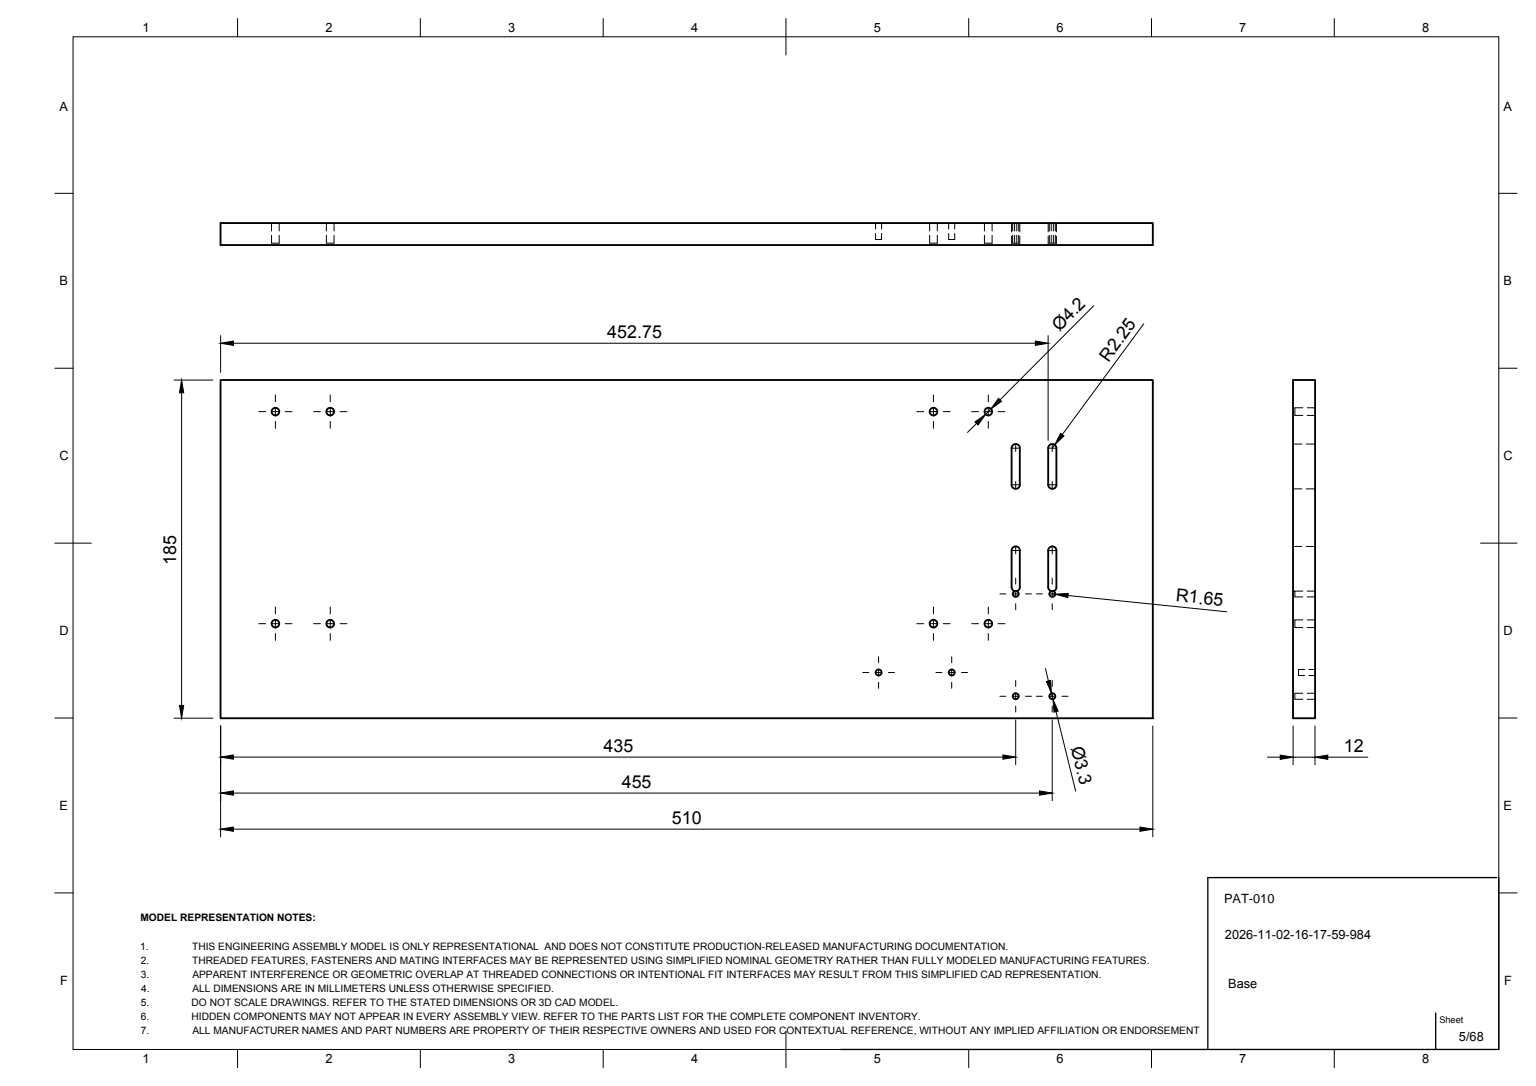
ISO-10303-21;
HEADER;
/* Generated by software containing ST-Developer
 * from STEP Tools, Inc. (www.steptools.com) 
 */

FILE_DESCRIPTION(
/* description */ ('Belt conveyor head drive unit'),
/* implementation_level */ '2;1');

FILE_NAME(
/* name */ 'Base.step',
/* time_stamp */ '2026-10-28T03:26:19-07:00',
/* author */ (''),
/* organization */ (''),
/* preprocessor_version */ 'ST-DEVELOPER v20.2',
/* originating_system */ 'Autodesk Translation Framework v15.17.0.0',
/* authorisation */ '');

FILE_SCHEMA (('AUTOMOTIVE_DESIGN { 1 0 10303 214 3 1 1 }'));
ENDSEC;

DATA;
#10=MECHANICAL_DESIGN_GEOMETRIC_PRESENTATION_REPRESENTATION('',(#847),#27069);
#709=SHAPE_REPRESENTATION_RELATIONSHIP('SRR','None',#27353,#778);
#778=ADVANCED_BREP_SHAPE_REPRESENTATION('',(#932),#26995);
#847=STYLED_ITEM('',(#27776),#932);
#932=MANIFOLD_SOLID_BREP('Body1',#13712);
#1012=FACE_BOUND('',#2456,.T.);
#1013=FACE_BOUND('',#2457,.T.);
#1014=FACE_BOUND('',#2458,.T.);
#1015=FACE_BOUND('',#2459,.T.);
#1016=FACE_BOUND('',#2487,.T.);
#1017=FACE_BOUND('',#2488,.T.);
#1018=FACE_BOUND('',#2489,.T.);
#1019=FACE_BOUND('',#2490,.T.);
#1020=FACE_BOUND('',#2491,.T.);
#1021=FACE_BOUND('',#2492,.T.);
#1022=FACE_BOUND('',#2493,.T.);
#1023=FACE_BOUND('',#2494,.T.);
#1024=FACE_BOUND('',#2495,.T.);
#1025=FACE_BOUND('',#2496,.T.);
#1026=FACE_BOUND('',#2497,.T.);
#1027=FACE_BOUND('',#2498,.T.);
#1028=FACE_BOUND('',#2499,.T.);
#1029=FACE_BOUND('',#2500,.T.);
#1030=FACE_BOUND('',#2501,.T.);
#1031=FACE_BOUND('',#2502,.T.);
#1277=PLANE('',#14568);
#1278=PLANE('',#14572);
#1279=PLANE('',#14576);
#1280=PLANE('',#14580);
#1281=PLANE('',#14584);
#1282=PLANE('',#14588);
#1283=PLANE('',#14592);
#1284=PLANE('',#14596);
#1285=PLANE('',#14600);
#1286=PLANE('',#14604);
#1287=PLANE('',#14611);
#1288=PLANE('',#14618);
#1289=PLANE('',#14619);
#1290=PLANE('',#14624);
#1291=PLANE('',#14625);
#1292=PLANE('',#14632);
#1293=PLANE('',#14633);
#1294=PLANE('',#14640);
#1295=PLANE('',#14641);
#1296=PLANE('',#14645);
#1297=PLANE('',#14649);
#1298=PLANE('',#14653);
#1299=PLANE('',#14657);
#1300=PLANE('',#14658);
#1301=PLANE('',#14659);
#1302=PLANE('',#14660);
#1303=PLANE('',#14661);
#1304=PLANE('',#14662);
#1633=FACE_OUTER_BOUND('',#2433,.T.);
#1634=FACE_OUTER_BOUND('',#2434,.T.);
#1635=FACE_OUTER_BOUND('',#2435,.T.);
#1636=FACE_OUTER_BOUND('',#2436,.T.);
#1637=FACE_OUTER_BOUND('',#2437,.T.);
#1638=FACE_OUTER_BOUND('',#2438,.T.);
#1639=FACE_OUTER_BOUND('',#2439,.T.);
#1640=FACE_OUTER_BOUND('',#2440,.T.);
#1641=FACE_OUTER_BOUND('',#2441,.T.);
#1642=FACE_OUTER_BOUND('',#2442,.T.);
#1643=FACE_OUTER_BOUND('',#2443,.T.);
#1644=FACE_OUTER_BOUND('',#2444,.T.);
#1645=FACE_OUTER_BOUND('',#2445,.T.);
#1646=FACE_OUTER_BOUND('',#2446,.T.);
#1647=FACE_OUTER_BOUND('',#2447,.T.);
#1648=FACE_OUTER_BOUND('',#2448,.T.);
#1649=FACE_OUTER_BOUND('',#2449,.T.);
#1650=FACE_OUTER_BOUND('',#2450,.T.);
#1651=FACE_OUTER_BOUND('',#2451,.T.);
#1652=FACE_OUTER_BOUND('',#2452,.T.);
#1653=FACE_OUTER_BOUND('',#2453,.T.);
#1654=FACE_OUTER_BOUND('',#2454,.T.);
#1655=FACE_OUTER_BOUND('',#2455,.T.);
#1656=FACE_OUTER_BOUND('',#2460,.T.);
#1657=FACE_OUTER_BOUND('',#2461,.T.);
#1658=FACE_OUTER_BOUND('',#2462,.T.);
#1659=FACE_OUTER_BOUND('',#2463,.T.);
#1660=FACE_OUTER_BOUND('',#2464,.T.);
#1661=FACE_OUTER_BOUND('',#2465,.T.);
#1662=FACE_OUTER_BOUND('',#2466,.T.);
#1663=FACE_OUTER_BOUND('',#2467,.T.);
#1664=FACE_OUTER_BOUND('',#2468,.T.);
#1665=FACE_OUTER_BOUND('',#2469,.T.);
#1666=FACE_OUTER_BOUND('',#2470,.T.);
#1667=FACE_OUTER_BOUND('',#2471,.T.);
#1668=FACE_OUTER_BOUND('',#2472,.T.);
#1669=FACE_OUTER_BOUND('',#2473,.T.);
#1670=FACE_OUTER_BOUND('',#2474,.T.);
#1671=FACE_OUTER_BOUND('',#2475,.T.);
#1672=FACE_OUTER_BOUND('',#2476,.T.);
#1673=FACE_OUTER_BOUND('',#2477,.T.);
#1674=FACE_OUTER_BOUND('',#2478,.T.);
#1675=FACE_OUTER_BOUND('',#2479,.T.);
#1676=FACE_OUTER_BOUND('',#2480,.T.);
#1677=FACE_OUTER_BOUND('',#2481,.T.);
#1678=FACE_OUTER_BOUND('',#2482,.T.);
#1679=FACE_OUTER_BOUND('',#2483,.T.);
#1680=FACE_OUTER_BOUND('',#2484,.T.);
#1681=FACE_OUTER_BOUND('',#2485,.T.);
#1682=FACE_OUTER_BOUND('',#2486,.T.);
#2433=EDGE_LOOP('',(#8958,#8959,#8960,#8961));
#2434=EDGE_LOOP('',(#8962));
#2435=EDGE_LOOP('',(#8963,#8964,#8965,#8966));
#2436=EDGE_LOOP('',(#8967));
#2437=EDGE_LOOP('',(#8968,#8969,#8970,#8971));
#2438=EDGE_LOOP('',(#8972));
#2439=EDGE_LOOP('',(#8973,#8974,#8975,#8976));
#2440=EDGE_LOOP('',(#8977));
#2441=EDGE_LOOP('',(#8978,#8979,#8980,#8981));
#2442=EDGE_LOOP('',(#8982));
#2443=EDGE_LOOP('',(#8983,#8984,#8985,#8986));
#2444=EDGE_LOOP('',(#8987));
#2445=EDGE_LOOP('',(#8988,#8989,#8990,#8991));
#2446=EDGE_LOOP('',(#8992));
#2447=EDGE_LOOP('',(#8993,#8994,#8995,#8996));
#2448=EDGE_LOOP('',(#8997));
#2449=EDGE_LOOP('',(#8998,#8999,#9000,#9001));
#2450=EDGE_LOOP('',(#9002));
#2451=EDGE_LOOP('',(#9003,#9004,#9005,#9006));
#2452=EDGE_LOOP('',(#9007));
#2453=EDGE_LOOP('',(#9008,#9009,#9010,#9011));
#2454=EDGE_LOOP('',(#9012,#9013,#9014,#9015));
#2455=EDGE_LOOP('',(#9016,#9017,#9018,#9019));
#2456=EDGE_LOOP('',(#9020,#9021,#9022,#9023));
#2457=EDGE_LOOP('',(#9024,#9025,#9026,#9027));
#2458=EDGE_LOOP('',(#9028,#9029,#9030,#9031));
#2459=EDGE_LOOP('',(#9032,#9033,#9034,#9035));
#2460=EDGE_LOOP('',(#9036,#9037,#9038,#9039));
#2461=EDGE_LOOP('',(#9040,#9041,#9042,#9043));
#2462=EDGE_LOOP('',(#9044,#9045,#9046,#9047));
#2463=EDGE_LOOP('',(#9048,#9049,#9050,#9051));
#2464=EDGE_LOOP('',(#9052,#9053,#9054,#9055));
#2465=EDGE_LOOP('',(#9056,#9057,#9058,#9059));
#2466=EDGE_LOOP('',(#9060,#9061,#9062,#9063,#9064,#9065,#9066,#9067));
#2467=EDGE_LOOP('',(#9068,#9069,#9070,#9071));
#2468=EDGE_LOOP('',(#9072,#9073,#9074,#9075));
#2469=EDGE_LOOP('',(#9076,#9077,#9078,#9079));
#2470=EDGE_LOOP('',(#9080,#9081,#9082,#9083,#9084,#9085,#9086,#9087));
#2471=EDGE_LOOP('',(#9088,#9089,#9090,#9091));
#2472=EDGE_LOOP('',(#9092,#9093,#9094,#9095));
#2473=EDGE_LOOP('',(#9096,#9097,#9098,#9099));
#2474=EDGE_LOOP('',(#9100,#9101,#9102,#9103));
#2475=EDGE_LOOP('',(#9104,#9105));
#2476=EDGE_LOOP('',(#9106,#9107,#9108,#9109));
#2477=EDGE_LOOP('',(#9110));
#2478=EDGE_LOOP('',(#9111,#9112,#9113,#9114));
#2479=EDGE_LOOP('',(#9115));
#2480=EDGE_LOOP('',(#9116,#9117,#9118,#9119));
#2481=EDGE_LOOP('',(#9120,#9121));
#2482=EDGE_LOOP('',(#9122,#9123,#9124,#9125));
#2483=EDGE_LOOP('',(#9126,#9127,#9128,#9129));
#2484=EDGE_LOOP('',(#9130,#9131,#9132,#9133));
#2485=EDGE_LOOP('',(#9134,#9135,#9136,#9137));
#2486=EDGE_LOOP('',(#9138,#9139,#9140,#9141));
#2487=EDGE_LOOP('',(#9142));
#2488=EDGE_LOOP('',(#9143));
#2489=EDGE_LOOP('',(#9144));
#2490=EDGE_LOOP('',(#9145));
#2491=EDGE_LOOP('',(#9146));
#2492=EDGE_LOOP('',(#9147));
#2493=EDGE_LOOP('',(#9148,#9149,#9150,#9151,#9152,#9153));
#2494=EDGE_LOOP('',(#9154,#9155,#9156,#9157,#9158,#9159));
#2495=EDGE_LOOP('',(#9160,#9161,#9162,#9163));
#2496=EDGE_LOOP('',(#9164,#9165,#9166,#9167));
#2497=EDGE_LOOP('',(#9168));
#2498=EDGE_LOOP('',(#9169));
#2499=EDGE_LOOP('',(#9170));
#2500=EDGE_LOOP('',(#9171));
#2501=EDGE_LOOP('',(#9172));
#2502=EDGE_LOOP('',(#9173));
#3498=LINE('',#20977,#4290);
#3499=LINE('',#20984,#4291);
#3500=LINE('',#20991,#4292);
#3501=LINE('',#20998,#4293);
#3502=LINE('',#21005,#4294);
#3503=LINE('',#21012,#4295);
#3504=LINE('',#21019,#4296);
#3505=LINE('',#21026,#4297);
#3506=LINE('',#21033,#4298);
#3507=LINE('',#21040,#4299);
#3508=LINE('',#21046,#4300);
#3509=LINE('',#21050,#4301);
#3510=LINE('',#21055,#4302);
#3511=LINE('',#21059,#4303);
#3512=LINE('',#21064,#4304);
#3513=LINE('',#21066,#4305);
#3514=LINE('',#21068,#4306);
#3515=LINE('',#21069,#4307);
#3516=LINE('',#21074,#4308);
#3517=LINE('',#21077,#4309);
#3518=LINE('',#21082,#4310);
#3519=LINE('',#21085,#4311);
#3520=LINE('',#21090,#4312);
#3521=LINE('',#21093,#4313);
#3522=LINE('',#21094,#4314);
#3523=LINE('',#21095,#4315);
#3524=LINE('',#21097,#4316);
#3525=LINE('',#21099,#4317);
#3526=LINE('',#21102,#4318);
#3527=LINE('',#21104,#4319);
#3528=LINE('',#21108,#4320);
#3529=LINE('',#21111,#4321);
#3530=LINE('',#21113,#4322);
#3531=LINE('',#21115,#4323);
#3532=LINE('',#21119,#4324);
#3533=LINE('',#21122,#4325);
#3534=LINE('',#21124,#4326);
#3535=LINE('',#21128,#4327);
#3536=LINE('',#21132,#4328);
#3537=LINE('',#21135,#4329);
#3538=LINE('',#21137,#4330);
#3539=LINE('',#21139,#4331);
#3540=LINE('',#21143,#4332);
#3541=LINE('',#21146,#4333);
#3542=LINE('',#21148,#4334);
#3543=LINE('',#21152,#4335);
#3544=LINE('',#21156,#4336);
#3545=LINE('',#21159,#4337);
#3546=LINE('',#21161,#4338);
#3547=LINE('',#21163,#4339);
#3548=LINE('',#21172,#4340);
#3549=LINE('',#21179,#4341);
#3550=LINE('',#21188,#4342);
#3551=LINE('',#21190,#4343);
#3552=LINE('',#21191,#4344);
#3553=LINE('',#21194,#4345);
#3554=LINE('',#21195,#4346);
#3555=LINE('',#21198,#4347);
#3556=LINE('',#21199,#4348);
#3557=LINE('',#21201,#4349);
#4290=VECTOR('',#16444,0.165);
#4291=VECTOR('',#16453,0.165);
#4292=VECTOR('',#16462,0.210000000000001);
#4293=VECTOR('',#16471,0.210000000000001);
#4294=VECTOR('',#16480,0.21);
#4295=VECTOR('',#16489,0.21);
#4296=VECTOR('',#16498,0.210000000000001);
#4297=VECTOR('',#16507,0.210000000000001);
#4298=VECTOR('',#16516,0.21);
#4299=VECTOR('',#16525,0.21);
#4300=VECTOR('',#16532,1.);
#4301=VECTOR('',#16535,1.);
#4302=VECTOR('',#16540,1.);
#4303=VECTOR('',#16543,1.);
#4304=VECTOR('',#16548,1.);
#4305=VECTOR('',#16549,1.);
#4306=VECTOR('',#16550,1.);
#4307=VECTOR('',#16551,1.);
#4308=VECTOR('',#16554,1.);
#4309=VECTOR('',#16557,1.);
#4310=VECTOR('',#16560,1.);
#4311=VECTOR('',#16563,1.);
#4312=VECTOR('',#16566,1.);
#4313=VECTOR('',#16569,1.);
#4314=VECTOR('',#16570,1.);
#4315=VECTOR('',#16571,1.);
#4316=VECTOR('',#16574,1.);
#4317=VECTOR('',#16577,1.);
#4318=VECTOR('',#16580,1.);
#4319=VECTOR('',#16581,1.);
#4320=VECTOR('',#16586,1.);
#4321=VECTOR('',#16589,1.);
#4322=VECTOR('',#16592,1.);
#4323=VECTOR('',#16595,1.);
#4324=VECTOR('',#16598,1.);
#4325=VECTOR('',#16601,1.);
#4326=VECTOR('',#16602,1.);
#4327=VECTOR('',#16605,1.);
#4328=VECTOR('',#16610,1.);
#4329=VECTOR('',#16613,1.);
#4330=VECTOR('',#16616,1.);
#4331=VECTOR('',#16619,1.);
#4332=VECTOR('',#16622,1.);
#4333=VECTOR('',#16625,1.);
#4334=VECTOR('',#16626,1.);
#4335=VECTOR('',#16629,1.);
#4336=VECTOR('',#16634,1.);
#4337=VECTOR('',#16637,1.);
#4338=VECTOR('',#16640,1.);
#4339=VECTOR('',#16643,1.);
#4340=VECTOR('',#16656,0.165);
#4341=VECTOR('',#16665,0.165);
#4342=VECTOR('',#16680,1.);
#4343=VECTOR('',#16681,1.);
#4344=VECTOR('',#16682,1.);
#4345=VECTOR('',#16685,1.);
#4346=VECTOR('',#16686,1.);
#4347=VECTOR('',#16689,1.);
#4348=VECTOR('',#16690,1.);
#4349=VECTOR('',#16693,1.);
#5082=CIRCLE('',#14566,0.165);
#5083=CIRCLE('',#14567,0.165);
#5084=CIRCLE('',#14570,0.165);
#5085=CIRCLE('',#14571,0.165);
#5086=CIRCLE('',#14574,0.210000000000001);
#5087=CIRCLE('',#14575,0.210000000000001);
#5088=CIRCLE('',#14578,0.210000000000001);
#5089=CIRCLE('',#14579,0.210000000000001);
#5090=CIRCLE('',#14582,0.21);
#5091=CIRCLE('',#14583,0.21);
#5092=CIRCLE('',#14586,0.21);
#5093=CIRCLE('',#14587,0.21);
#5094=CIRCLE('',#14590,0.210000000000001);
#5095=CIRCLE('',#14591,0.210000000000001);
#5096=CIRCLE('',#14594,0.210000000000001);
#5097=CIRCLE('',#14595,0.210000000000001);
#5098=CIRCLE('',#14598,0.21);
#5099=CIRCLE('',#14599,0.21);
#5100=CIRCLE('',#14602,0.21);
#5101=CIRCLE('',#14603,0.21);
#5102=CIRCLE('',#14606,0.225);
#5103=CIRCLE('',#14607,0.225);
#5104=CIRCLE('',#14609,0.225);
#5105=CIRCLE('',#14610,0.225);
#5106=CIRCLE('',#14612,0.225);
#5107=CIRCLE('',#14613,0.225);
#5108=CIRCLE('',#14614,0.225);
#5109=CIRCLE('',#14615,0.225);
#5110=CIRCLE('',#14616,0.225);
#5111=CIRCLE('',#14617,0.225);
#5112=CIRCLE('',#14621,0.225);
#5113=CIRCLE('',#14623,0.225);
#5114=CIRCLE('',#14627,0.225);
#5115=CIRCLE('',#14628,0.225);
#5116=CIRCLE('',#14629,0.225);
#5117=CIRCLE('',#14631,0.225);
#5118=CIRCLE('',#14635,0.225);
#5119=CIRCLE('',#14636,0.225);
#5120=CIRCLE('',#14637,0.225);
#5121=CIRCLE('',#14639,0.225);
#5122=CIRCLE('',#14643,0.165);
#5123=CIRCLE('',#14644,0.165);
#5124=CIRCLE('',#14647,0.165);
#5125=CIRCLE('',#14648,0.165);
#5126=CIRCLE('',#14651,0.165);
#5127=CIRCLE('',#14652,0.165);
#5128=CIRCLE('',#14655,0.165);
#5129=CIRCLE('',#14656,0.165);
#5953=VERTEX_POINT('',#20974);
#5954=VERTEX_POINT('',#20976);
#5955=VERTEX_POINT('',#20981);
#5956=VERTEX_POINT('',#20983);
#5957=VERTEX_POINT('',#20988);
#5958=VERTEX_POINT('',#20990);
#5959=VERTEX_POINT('',#20995);
#5960=VERTEX_POINT('',#20997);
#5961=VERTEX_POINT('',#21002);
#5962=VERTEX_POINT('',#21004);
#5963=VERTEX_POINT('',#21009);
#5964=VERTEX_POINT('',#21011);
#5965=VERTEX_POINT('',#21016);
#5966=VERTEX_POINT('',#21018);
#5967=VERTEX_POINT('',#21023);
#5968=VERTEX_POINT('',#21025);
#5969=VERTEX_POINT('',#21030);
#5970=VERTEX_POINT('',#21032);
#5971=VERTEX_POINT('',#21037);
#5972=VERTEX_POINT('',#21039);
#5973=VERTEX_POINT('',#21044);
#5974=VERTEX_POINT('',#21045);
#5975=VERTEX_POINT('',#21047);
#5976=VERTEX_POINT('',#21049);
#5977=VERTEX_POINT('',#21053);
#5978=VERTEX_POINT('',#21054);
#5979=VERTEX_POINT('',#21056);
#5980=VERTEX_POINT('',#21058);
#5981=VERTEX_POINT('',#21062);
#5982=VERTEX_POINT('',#21063);
#5983=VERTEX_POINT('',#21065);
#5984=VERTEX_POINT('',#21067);
#5985=VERTEX_POINT('',#21070);
#5986=VERTEX_POINT('',#21071);
#5987=VERTEX_POINT('',#21073);
#5988=VERTEX_POINT('',#21075);
#5989=VERTEX_POINT('',#21078);
#5990=VERTEX_POINT('',#21079);
#5991=VERTEX_POINT('',#21081);
#5992=VERTEX_POINT('',#21083);
#5993=VERTEX_POINT('',#21086);
#5994=VERTEX_POINT('',#21087);
#5995=VERTEX_POINT('',#21089);
#5996=VERTEX_POINT('',#21091);
#5997=VERTEX_POINT('',#21101);
#5998=VERTEX_POINT('',#21103);
#5999=VERTEX_POINT('',#21107);
#6000=VERTEX_POINT('',#21109);
#6001=VERTEX_POINT('',#21117);
#6002=VERTEX_POINT('',#21118);
#6003=VERTEX_POINT('',#21120);
#6004=VERTEX_POINT('',#21123);
#6005=VERTEX_POINT('',#21125);
#6006=VERTEX_POINT('',#21127);
#6007=VERTEX_POINT('',#21131);
#6008=VERTEX_POINT('',#21133);
#6009=VERTEX_POINT('',#21141);
#6010=VERTEX_POINT('',#21142);
#6011=VERTEX_POINT('',#21144);
#6012=VERTEX_POINT('',#21147);
#6013=VERTEX_POINT('',#21149);
#6014=VERTEX_POINT('',#21151);
#6015=VERTEX_POINT('',#21155);
#6016=VERTEX_POINT('',#21157);
#6017=VERTEX_POINT('',#21169);
#6018=VERTEX_POINT('',#21171);
#6019=VERTEX_POINT('',#21176);
#6020=VERTEX_POINT('',#21178);
#6021=VERTEX_POINT('',#21187);
#6022=VERTEX_POINT('',#21189);
#6023=VERTEX_POINT('',#21193);
#6024=VERTEX_POINT('',#21197);
#7171=EDGE_CURVE('',#5953,#5953,#5082,.T.);
#7172=EDGE_CURVE('',#5953,#5954,#3498,.T.);
#7173=EDGE_CURVE('',#5954,#5954,#5083,.T.);
#7174=EDGE_CURVE('',#5955,#5955,#5084,.T.);
#7175=EDGE_CURVE('',#5955,#5956,#3499,.T.);
#7176=EDGE_CURVE('',#5956,#5956,#5085,.T.);
#7177=EDGE_CURVE('',#5957,#5957,#5086,.T.);
#7178=EDGE_CURVE('',#5957,#5958,#3500,.T.);
#7179=EDGE_CURVE('',#5958,#5958,#5087,.T.);
#7180=EDGE_CURVE('',#5959,#5959,#5088,.T.);
#7181=EDGE_CURVE('',#5959,#5960,#3501,.T.);
#7182=EDGE_CURVE('',#5960,#5960,#5089,.T.);
#7183=EDGE_CURVE('',#5961,#5961,#5090,.T.);
#7184=EDGE_CURVE('',#5961,#5962,#3502,.T.);
#7185=EDGE_CURVE('',#5962,#5962,#5091,.T.);
#7186=EDGE_CURVE('',#5963,#5963,#5092,.T.);
#7187=EDGE_CURVE('',#5963,#5964,#3503,.T.);
#7188=EDGE_CURVE('',#5964,#5964,#5093,.T.);
#7189=EDGE_CURVE('',#5965,#5965,#5094,.T.);
#7190=EDGE_CURVE('',#5965,#5966,#3504,.T.);
#7191=EDGE_CURVE('',#5966,#5966,#5095,.T.);
#7192=EDGE_CURVE('',#5967,#5967,#5096,.T.);
#7193=EDGE_CURVE('',#5967,#5968,#3505,.T.);
#7194=EDGE_CURVE('',#5968,#5968,#5097,.T.);
#7195=EDGE_CURVE('',#5969,#5969,#5098,.T.);
#7196=EDGE_CURVE('',#5969,#5970,#3506,.T.);
#7197=EDGE_CURVE('',#5970,#5970,#5099,.T.);
#7198=EDGE_CURVE('',#5971,#5971,#5100,.T.);
#7199=EDGE_CURVE('',#5971,#5972,#3507,.T.);
#7200=EDGE_CURVE('',#5972,#5972,#5101,.T.);
#7201=EDGE_CURVE('',#5973,#5974,#3508,.T.);
#7202=EDGE_CURVE('',#5975,#5973,#5102,.T.);
#7203=EDGE_CURVE('',#5975,#5976,#3509,.T.);
#7204=EDGE_CURVE('',#5974,#5976,#5103,.T.);
#7205=EDGE_CURVE('',#5977,#5978,#3510,.T.);
#7206=EDGE_CURVE('',#5979,#5978,#5104,.T.);
#7207=EDGE_CURVE('',#5980,#5979,#3511,.T.);
#7208=EDGE_CURVE('',#5977,#5980,#5105,.T.);
#7209=EDGE_CURVE('',#5981,#5982,#3512,.T.);
#7210=EDGE_CURVE('',#5983,#5981,#3513,.T.);
#7211=EDGE_CURVE('',#5984,#5983,#3514,.T.);
#7212=EDGE_CURVE('',#5982,#5984,#3515,.T.);
#7213=EDGE_CURVE('',#5985,#5986,#5106,.T.);
#7214=EDGE_CURVE('',#5986,#5987,#3516,.T.);
#7215=EDGE_CURVE('',#5987,#5988,#5107,.T.);
#7216=EDGE_CURVE('',#5988,#5985,#3517,.T.);
#7217=EDGE_CURVE('',#5989,#5990,#5108,.T.);
#7218=EDGE_CURVE('',#5990,#5991,#3518,.T.);
#7219=EDGE_CURVE('',#5991,#5992,#5109,.T.);
#7220=EDGE_CURVE('',#5992,#5989,#3519,.T.);
#7221=EDGE_CURVE('',#5993,#5994,#5110,.T.);
#7222=EDGE_CURVE('',#5994,#5995,#3520,.T.);
#7223=EDGE_CURVE('',#5995,#5996,#5111,.T.);
#7224=EDGE_CURVE('',#5996,#5993,#3521,.T.);
#7225=EDGE_CURVE('',#5973,#5977,#3522,.T.);
#7226=EDGE_CURVE('',#5980,#5975,#3523,.T.);
#7227=EDGE_CURVE('',#5976,#5979,#3524,.T.);
#7228=EDGE_CURVE('',#5978,#5974,#3525,.T.);
#7229=EDGE_CURVE('',#5986,#5997,#3526,.T.);
#7230=EDGE_CURVE('',#5985,#5998,#3527,.T.);
#7231=EDGE_CURVE('',#5997,#5998,#5112,.T.);
#7232=EDGE_CURVE('',#5987,#5999,#3528,.T.);
#7233=EDGE_CURVE('',#6000,#5999,#5113,.T.);
#7234=EDGE_CURVE('',#5988,#6000,#3529,.T.);
#7235=EDGE_CURVE('',#5998,#6000,#3530,.T.);
#7236=EDGE_CURVE('',#5999,#5997,#3531,.T.);
#7237=EDGE_CURVE('',#6001,#6002,#3532,.T.);
#7238=EDGE_CURVE('',#6003,#6001,#5114,.T.);
#7239=EDGE_CURVE('',#5994,#6003,#3533,.T.);
#7240=EDGE_CURVE('',#5993,#6004,#3534,.T.);
#7241=EDGE_CURVE('',#6005,#6004,#5115,.T.);
#7242=EDGE_CURVE('',#6006,#6005,#3535,.T.);
#7243=EDGE_CURVE('',#6002,#6006,#5116,.T.);
#7244=EDGE_CURVE('',#5995,#6007,#3536,.T.);
#7245=EDGE_CURVE('',#6008,#6007,#5117,.T.);
#7246=EDGE_CURVE('',#5996,#6008,#3537,.T.);
#7247=EDGE_CURVE('',#6004,#6008,#3538,.T.);
#7248=EDGE_CURVE('',#6007,#6003,#3539,.T.);
#7249=EDGE_CURVE('',#6009,#6010,#3540,.T.);
#7250=EDGE_CURVE('',#6011,#6009,#5118,.T.);
#7251=EDGE_CURVE('',#5990,#6011,#3541,.T.);
#7252=EDGE_CURVE('',#5989,#6012,#3542,.T.);
#7253=EDGE_CURVE('',#6013,#6012,#5119,.T.);
#7254=EDGE_CURVE('',#6014,#6013,#3543,.T.);
#7255=EDGE_CURVE('',#6010,#6014,#5120,.T.);
#7256=EDGE_CURVE('',#5991,#6015,#3544,.T.);
#7257=EDGE_CURVE('',#6016,#6015,#5121,.T.);
#7258=EDGE_CURVE('',#5992,#6016,#3545,.T.);
#7259=EDGE_CURVE('',#6012,#6016,#3546,.T.);
#7260=EDGE_CURVE('',#6015,#6011,#3547,.T.);
#7261=EDGE_CURVE('',#6009,#6013,#5122,.T.);
#7262=EDGE_CURVE('',#6014,#6010,#5123,.T.);
#7263=EDGE_CURVE('',#6017,#6017,#5124,.T.);
#7264=EDGE_CURVE('',#6017,#6018,#3548,.T.);
#7265=EDGE_CURVE('',#6018,#6018,#5125,.T.);
#7266=EDGE_CURVE('',#6019,#6019,#5126,.T.);
#7267=EDGE_CURVE('',#6019,#6020,#3549,.T.);
#7268=EDGE_CURVE('',#6020,#6020,#5127,.T.);
#7269=EDGE_CURVE('',#6001,#6005,#5128,.T.);
#7270=EDGE_CURVE('',#6006,#6002,#5129,.T.);
#7271=EDGE_CURVE('',#5981,#6021,#3550,.T.);
#7272=EDGE_CURVE('',#6022,#6021,#3551,.T.);
#7273=EDGE_CURVE('',#5983,#6022,#3552,.T.);
#7274=EDGE_CURVE('',#6023,#6022,#3553,.T.);
#7275=EDGE_CURVE('',#5984,#6023,#3554,.T.);
#7276=EDGE_CURVE('',#6024,#6023,#3555,.T.);
#7277=EDGE_CURVE('',#5982,#6024,#3556,.T.);
#7278=EDGE_CURVE('',#6021,#6024,#3557,.T.);
#8958=ORIENTED_EDGE('',*,*,#7171,.F.);
#8959=ORIENTED_EDGE('',*,*,#7172,.T.);
#8960=ORIENTED_EDGE('',*,*,#7173,.F.);
#8961=ORIENTED_EDGE('',*,*,#7172,.F.);
#8962=ORIENTED_EDGE('',*,*,#7171,.T.);
#8963=ORIENTED_EDGE('',*,*,#7174,.F.);
#8964=ORIENTED_EDGE('',*,*,#7175,.T.);
#8965=ORIENTED_EDGE('',*,*,#7176,.F.);
#8966=ORIENTED_EDGE('',*,*,#7175,.F.);
#8967=ORIENTED_EDGE('',*,*,#7174,.T.);
#8968=ORIENTED_EDGE('',*,*,#7177,.F.);
#8969=ORIENTED_EDGE('',*,*,#7178,.T.);
#8970=ORIENTED_EDGE('',*,*,#7179,.F.);
#8971=ORIENTED_EDGE('',*,*,#7178,.F.);
#8972=ORIENTED_EDGE('',*,*,#7177,.T.);
#8973=ORIENTED_EDGE('',*,*,#7180,.F.);
#8974=ORIENTED_EDGE('',*,*,#7181,.T.);
#8975=ORIENTED_EDGE('',*,*,#7182,.F.);
#8976=ORIENTED_EDGE('',*,*,#7181,.F.);
#8977=ORIENTED_EDGE('',*,*,#7180,.T.);
#8978=ORIENTED_EDGE('',*,*,#7183,.F.);
#8979=ORIENTED_EDGE('',*,*,#7184,.T.);
#8980=ORIENTED_EDGE('',*,*,#7185,.F.);
#8981=ORIENTED_EDGE('',*,*,#7184,.F.);
#8982=ORIENTED_EDGE('',*,*,#7183,.T.);
#8983=ORIENTED_EDGE('',*,*,#7186,.F.);
#8984=ORIENTED_EDGE('',*,*,#7187,.T.);
#8985=ORIENTED_EDGE('',*,*,#7188,.F.);
#8986=ORIENTED_EDGE('',*,*,#7187,.F.);
#8987=ORIENTED_EDGE('',*,*,#7186,.T.);
#8988=ORIENTED_EDGE('',*,*,#7189,.F.);
#8989=ORIENTED_EDGE('',*,*,#7190,.T.);
#8990=ORIENTED_EDGE('',*,*,#7191,.F.);
#8991=ORIENTED_EDGE('',*,*,#7190,.F.);
#8992=ORIENTED_EDGE('',*,*,#7189,.T.);
#8993=ORIENTED_EDGE('',*,*,#7192,.F.);
#8994=ORIENTED_EDGE('',*,*,#7193,.T.);
#8995=ORIENTED_EDGE('',*,*,#7194,.F.);
#8996=ORIENTED_EDGE('',*,*,#7193,.F.);
#8997=ORIENTED_EDGE('',*,*,#7192,.T.);
#8998=ORIENTED_EDGE('',*,*,#7195,.F.);
#8999=ORIENTED_EDGE('',*,*,#7196,.T.);
#9000=ORIENTED_EDGE('',*,*,#7197,.F.);
#9001=ORIENTED_EDGE('',*,*,#7196,.F.);
#9002=ORIENTED_EDGE('',*,*,#7195,.T.);
#9003=ORIENTED_EDGE('',*,*,#7198,.F.);
#9004=ORIENTED_EDGE('',*,*,#7199,.T.);
#9005=ORIENTED_EDGE('',*,*,#7200,.F.);
#9006=ORIENTED_EDGE('',*,*,#7199,.F.);
#9007=ORIENTED_EDGE('',*,*,#7198,.T.);
#9008=ORIENTED_EDGE('',*,*,#7201,.F.);
#9009=ORIENTED_EDGE('',*,*,#7202,.F.);
#9010=ORIENTED_EDGE('',*,*,#7203,.T.);
#9011=ORIENTED_EDGE('',*,*,#7204,.F.);
#9012=ORIENTED_EDGE('',*,*,#7205,.T.);
#9013=ORIENTED_EDGE('',*,*,#7206,.F.);
#9014=ORIENTED_EDGE('',*,*,#7207,.F.);
#9015=ORIENTED_EDGE('',*,*,#7208,.F.);
#9016=ORIENTED_EDGE('',*,*,#7209,.F.);
#9017=ORIENTED_EDGE('',*,*,#7210,.F.);
#9018=ORIENTED_EDGE('',*,*,#7211,.F.);
#9019=ORIENTED_EDGE('',*,*,#7212,.F.);
#9020=ORIENTED_EDGE('',*,*,#7213,.T.);
#9021=ORIENTED_EDGE('',*,*,#7214,.T.);
#9022=ORIENTED_EDGE('',*,*,#7215,.T.);
#9023=ORIENTED_EDGE('',*,*,#7216,.T.);
#9024=ORIENTED_EDGE('',*,*,#7217,.T.);
#9025=ORIENTED_EDGE('',*,*,#7218,.T.);
#9026=ORIENTED_EDGE('',*,*,#7219,.T.);
#9027=ORIENTED_EDGE('',*,*,#7220,.T.);
#9028=ORIENTED_EDGE('',*,*,#7221,.T.);
#9029=ORIENTED_EDGE('',*,*,#7222,.T.);
#9030=ORIENTED_EDGE('',*,*,#7223,.T.);
#9031=ORIENTED_EDGE('',*,*,#7224,.T.);
#9032=ORIENTED_EDGE('',*,*,#7202,.T.);
#9033=ORIENTED_EDGE('',*,*,#7225,.T.);
#9034=ORIENTED_EDGE('',*,*,#7208,.T.);
#9035=ORIENTED_EDGE('',*,*,#7226,.T.);
#9036=ORIENTED_EDGE('',*,*,#7227,.F.);
#9037=ORIENTED_EDGE('',*,*,#7203,.F.);
#9038=ORIENTED_EDGE('',*,*,#7226,.F.);
#9039=ORIENTED_EDGE('',*,*,#7207,.T.);
#9040=ORIENTED_EDGE('',*,*,#7225,.F.);
#9041=ORIENTED_EDGE('',*,*,#7201,.T.);
#9042=ORIENTED_EDGE('',*,*,#7228,.F.);
#9043=ORIENTED_EDGE('',*,*,#7205,.F.);
#9044=ORIENTED_EDGE('',*,*,#7229,.F.);
#9045=ORIENTED_EDGE('',*,*,#7213,.F.);
#9046=ORIENTED_EDGE('',*,*,#7230,.T.);
#9047=ORIENTED_EDGE('',*,*,#7231,.F.);
#9048=ORIENTED_EDGE('',*,*,#7232,.T.);
#9049=ORIENTED_EDGE('',*,*,#7233,.F.);
#9050=ORIENTED_EDGE('',*,*,#7234,.F.);
#9051=ORIENTED_EDGE('',*,*,#7215,.F.);
#9052=ORIENTED_EDGE('',*,*,#7235,.F.);
#9053=ORIENTED_EDGE('',*,*,#7230,.F.);
#9054=ORIENTED_EDGE('',*,*,#7216,.F.);
#9055=ORIENTED_EDGE('',*,*,#7234,.T.);
#9056=ORIENTED_EDGE('',*,*,#7214,.F.);
#9057=ORIENTED_EDGE('',*,*,#7229,.T.);
#9058=ORIENTED_EDGE('',*,*,#7236,.F.);
#9059=ORIENTED_EDGE('',*,*,#7232,.F.);
#9060=ORIENTED_EDGE('',*,*,#7237,.F.);
#9061=ORIENTED_EDGE('',*,*,#7238,.F.);
#9062=ORIENTED_EDGE('',*,*,#7239,.F.);
#9063=ORIENTED_EDGE('',*,*,#7221,.F.);
#9064=ORIENTED_EDGE('',*,*,#7240,.T.);
#9065=ORIENTED_EDGE('',*,*,#7241,.F.);
#9066=ORIENTED_EDGE('',*,*,#7242,.F.);
#9067=ORIENTED_EDGE('',*,*,#7243,.F.);
#9068=ORIENTED_EDGE('',*,*,#7244,.T.);
#9069=ORIENTED_EDGE('',*,*,#7245,.F.);
#9070=ORIENTED_EDGE('',*,*,#7246,.F.);
#9071=ORIENTED_EDGE('',*,*,#7223,.F.);
#9072=ORIENTED_EDGE('',*,*,#7247,.F.);
#9073=ORIENTED_EDGE('',*,*,#7240,.F.);
#9074=ORIENTED_EDGE('',*,*,#7224,.F.);
#9075=ORIENTED_EDGE('',*,*,#7246,.T.);
#9076=ORIENTED_EDGE('',*,*,#7222,.F.);
#9077=ORIENTED_EDGE('',*,*,#7239,.T.);
#9078=ORIENTED_EDGE('',*,*,#7248,.F.);
#9079=ORIENTED_EDGE('',*,*,#7244,.F.);
#9080=ORIENTED_EDGE('',*,*,#7249,.F.);
#9081=ORIENTED_EDGE('',*,*,#7250,.F.);
#9082=ORIENTED_EDGE('',*,*,#7251,.F.);
#9083=ORIENTED_EDGE('',*,*,#7217,.F.);
#9084=ORIENTED_EDGE('',*,*,#7252,.T.);
#9085=ORIENTED_EDGE('',*,*,#7253,.F.);
#9086=ORIENTED_EDGE('',*,*,#7254,.F.);
#9087=ORIENTED_EDGE('',*,*,#7255,.F.);
#9088=ORIENTED_EDGE('',*,*,#7256,.T.);
#9089=ORIENTED_EDGE('',*,*,#7257,.F.);
#9090=ORIENTED_EDGE('',*,*,#7258,.F.);
#9091=ORIENTED_EDGE('',*,*,#7219,.F.);
#9092=ORIENTED_EDGE('',*,*,#7259,.F.);
#9093=ORIENTED_EDGE('',*,*,#7252,.F.);
#9094=ORIENTED_EDGE('',*,*,#7220,.F.);
#9095=ORIENTED_EDGE('',*,*,#7258,.T.);
#9096=ORIENTED_EDGE('',*,*,#7218,.F.);
#9097=ORIENTED_EDGE('',*,*,#7251,.T.);
#9098=ORIENTED_EDGE('',*,*,#7260,.F.);
#9099=ORIENTED_EDGE('',*,*,#7256,.F.);
#9100=ORIENTED_EDGE('',*,*,#7254,.T.);
#9101=ORIENTED_EDGE('',*,*,#7261,.F.);
#9102=ORIENTED_EDGE('',*,*,#7249,.T.);
#9103=ORIENTED_EDGE('',*,*,#7262,.F.);
#9104=ORIENTED_EDGE('',*,*,#7255,.T.);
#9105=ORIENTED_EDGE('',*,*,#7262,.T.);
#9106=ORIENTED_EDGE('',*,*,#7263,.F.);
#9107=ORIENTED_EDGE('',*,*,#7264,.T.);
#9108=ORIENTED_EDGE('',*,*,#7265,.F.);
#9109=ORIENTED_EDGE('',*,*,#7264,.F.);
#9110=ORIENTED_EDGE('',*,*,#7263,.T.);
#9111=ORIENTED_EDGE('',*,*,#7266,.F.);
#9112=ORIENTED_EDGE('',*,*,#7267,.T.);
#9113=ORIENTED_EDGE('',*,*,#7268,.F.);
#9114=ORIENTED_EDGE('',*,*,#7267,.F.);
#9115=ORIENTED_EDGE('',*,*,#7266,.T.);
#9116=ORIENTED_EDGE('',*,*,#7242,.T.);
#9117=ORIENTED_EDGE('',*,*,#7269,.F.);
#9118=ORIENTED_EDGE('',*,*,#7237,.T.);
#9119=ORIENTED_EDGE('',*,*,#7270,.F.);
#9120=ORIENTED_EDGE('',*,*,#7243,.T.);
#9121=ORIENTED_EDGE('',*,*,#7270,.T.);
#9122=ORIENTED_EDGE('',*,*,#7210,.T.);
#9123=ORIENTED_EDGE('',*,*,#7271,.T.);
#9124=ORIENTED_EDGE('',*,*,#7272,.F.);
#9125=ORIENTED_EDGE('',*,*,#7273,.F.);
#9126=ORIENTED_EDGE('',*,*,#7211,.T.);
#9127=ORIENTED_EDGE('',*,*,#7273,.T.);
#9128=ORIENTED_EDGE('',*,*,#7274,.F.);
#9129=ORIENTED_EDGE('',*,*,#7275,.F.);
#9130=ORIENTED_EDGE('',*,*,#7212,.T.);
#9131=ORIENTED_EDGE('',*,*,#7275,.T.);
#9132=ORIENTED_EDGE('',*,*,#7276,.F.);
#9133=ORIENTED_EDGE('',*,*,#7277,.F.);
#9134=ORIENTED_EDGE('',*,*,#7209,.T.);
#9135=ORIENTED_EDGE('',*,*,#7277,.T.);
#9136=ORIENTED_EDGE('',*,*,#7278,.F.);
#9137=ORIENTED_EDGE('',*,*,#7271,.F.);
#9138=ORIENTED_EDGE('',*,*,#7278,.T.);
#9139=ORIENTED_EDGE('',*,*,#7276,.T.);
#9140=ORIENTED_EDGE('',*,*,#7274,.T.);
#9141=ORIENTED_EDGE('',*,*,#7272,.T.);
#9142=ORIENTED_EDGE('',*,*,#7176,.T.);
#9143=ORIENTED_EDGE('',*,*,#7182,.T.);
#9144=ORIENTED_EDGE('',*,*,#7188,.T.);
#9145=ORIENTED_EDGE('',*,*,#7194,.T.);
#9146=ORIENTED_EDGE('',*,*,#7268,.T.);
#9147=ORIENTED_EDGE('',*,*,#7265,.T.);
#9148=ORIENTED_EDGE('',*,*,#7253,.T.);
#9149=ORIENTED_EDGE('',*,*,#7259,.T.);
#9150=ORIENTED_EDGE('',*,*,#7257,.T.);
#9151=ORIENTED_EDGE('',*,*,#7260,.T.);
#9152=ORIENTED_EDGE('',*,*,#7250,.T.);
#9153=ORIENTED_EDGE('',*,*,#7261,.T.);
#9154=ORIENTED_EDGE('',*,*,#7241,.T.);
#9155=ORIENTED_EDGE('',*,*,#7247,.T.);
#9156=ORIENTED_EDGE('',*,*,#7245,.T.);
#9157=ORIENTED_EDGE('',*,*,#7248,.T.);
#9158=ORIENTED_EDGE('',*,*,#7238,.T.);
#9159=ORIENTED_EDGE('',*,*,#7269,.T.);
#9160=ORIENTED_EDGE('',*,*,#7231,.T.);
#9161=ORIENTED_EDGE('',*,*,#7235,.T.);
#9162=ORIENTED_EDGE('',*,*,#7233,.T.);
#9163=ORIENTED_EDGE('',*,*,#7236,.T.);
#9164=ORIENTED_EDGE('',*,*,#7204,.T.);
#9165=ORIENTED_EDGE('',*,*,#7227,.T.);
#9166=ORIENTED_EDGE('',*,*,#7206,.T.);
#9167=ORIENTED_EDGE('',*,*,#7228,.T.);
#9168=ORIENTED_EDGE('',*,*,#7200,.T.);
#9169=ORIENTED_EDGE('',*,*,#7197,.T.);
#9170=ORIENTED_EDGE('',*,*,#7191,.T.);
#9171=ORIENTED_EDGE('',*,*,#7185,.T.);
#9172=ORIENTED_EDGE('',*,*,#7179,.T.);
#9173=ORIENTED_EDGE('',*,*,#7173,.T.);
#12532=CYLINDRICAL_SURFACE('',#14565,0.165);
#12533=CYLINDRICAL_SURFACE('',#14569,0.165);
#12534=CYLINDRICAL_SURFACE('',#14573,0.210000000000001);
#12535=CYLINDRICAL_SURFACE('',#14577,0.210000000000001);
#12536=CYLINDRICAL_SURFACE('',#14581,0.21);
#12537=CYLINDRICAL_SURFACE('',#14585,0.21);
#12538=CYLINDRICAL_SURFACE('',#14589,0.210000000000001);
#12539=CYLINDRICAL_SURFACE('',#14593,0.210000000000001);
#12540=CYLINDRICAL_SURFACE('',#14597,0.21);
#12541=CYLINDRICAL_SURFACE('',#14601,0.21);
#12542=CYLINDRICAL_SURFACE('',#14605,0.225);
#12543=CYLINDRICAL_SURFACE('',#14608,0.225);
#12544=CYLINDRICAL_SURFACE('',#14620,0.225);
#12545=CYLINDRICAL_SURFACE('',#14622,0.225);
#12546=CYLINDRICAL_SURFACE('',#14626,0.225);
#12547=CYLINDRICAL_SURFACE('',#14630,0.225);
#12548=CYLINDRICAL_SURFACE('',#14634,0.225);
#12549=CYLINDRICAL_SURFACE('',#14638,0.225);
#12550=CYLINDRICAL_SURFACE('',#14642,0.165);
#12551=CYLINDRICAL_SURFACE('',#14646,0.165);
#12552=CYLINDRICAL_SURFACE('',#14650,0.165);
#12553=CYLINDRICAL_SURFACE('',#14654,0.165);
#12912=ADVANCED_FACE('',(#1633),#12532,.F.);
#12913=ADVANCED_FACE('',(#1634),#1277,.T.);
#12914=ADVANCED_FACE('',(#1635),#12533,.F.);
#12915=ADVANCED_FACE('',(#1636),#1278,.T.);
#12916=ADVANCED_FACE('',(#1637),#12534,.F.);
#12917=ADVANCED_FACE('',(#1638),#1279,.T.);
#12918=ADVANCED_FACE('',(#1639),#12535,.F.);
#12919=ADVANCED_FACE('',(#1640),#1280,.T.);
#12920=ADVANCED_FACE('',(#1641),#12536,.F.);
#12921=ADVANCED_FACE('',(#1642),#1281,.T.);
#12922=ADVANCED_FACE('',(#1643),#12537,.F.);
#12923=ADVANCED_FACE('',(#1644),#1282,.T.);
#12924=ADVANCED_FACE('',(#1645),#12538,.F.);
#12925=ADVANCED_FACE('',(#1646),#1283,.T.);
#12926=ADVANCED_FACE('',(#1647),#12539,.F.);
#12927=ADVANCED_FACE('',(#1648),#1284,.T.);
#12928=ADVANCED_FACE('',(#1649),#12540,.F.);
#12929=ADVANCED_FACE('',(#1650),#1285,.T.);
#12930=ADVANCED_FACE('',(#1651),#12541,.F.);
#12931=ADVANCED_FACE('',(#1652),#1286,.T.);
#12932=ADVANCED_FACE('',(#1653),#12542,.F.);
#12933=ADVANCED_FACE('',(#1654),#12543,.F.);
#12934=ADVANCED_FACE('',(#1655,#1012,#1013,#1014,#1015),#1287,.F.);
#12935=ADVANCED_FACE('',(#1656),#1288,.F.);
#12936=ADVANCED_FACE('',(#1657),#1289,.F.);
#12937=ADVANCED_FACE('',(#1658),#12544,.F.);
#12938=ADVANCED_FACE('',(#1659),#12545,.F.);
#12939=ADVANCED_FACE('',(#1660),#1290,.F.);
#12940=ADVANCED_FACE('',(#1661),#1291,.F.);
#12941=ADVANCED_FACE('',(#1662),#12546,.F.);
#12942=ADVANCED_FACE('',(#1663),#12547,.F.);
#12943=ADVANCED_FACE('',(#1664),#1292,.F.);
#12944=ADVANCED_FACE('',(#1665),#1293,.F.);
#12945=ADVANCED_FACE('',(#1666),#12548,.F.);
#12946=ADVANCED_FACE('',(#1667),#12549,.F.);
#12947=ADVANCED_FACE('',(#1668),#1294,.F.);
#12948=ADVANCED_FACE('',(#1669),#1295,.F.);
#12949=ADVANCED_FACE('',(#1670),#12550,.F.);
#12950=ADVANCED_FACE('',(#1671),#1296,.T.);
#12951=ADVANCED_FACE('',(#1672),#12551,.F.);
#12952=ADVANCED_FACE('',(#1673),#1297,.T.);
#12953=ADVANCED_FACE('',(#1674),#12552,.F.);
#12954=ADVANCED_FACE('',(#1675),#1298,.T.);
#12955=ADVANCED_FACE('',(#1676),#12553,.F.);
#12956=ADVANCED_FACE('',(#1677),#1299,.T.);
#12957=ADVANCED_FACE('',(#1678),#1300,.T.);
#12958=ADVANCED_FACE('',(#1679),#1301,.T.);
#12959=ADVANCED_FACE('',(#1680),#1302,.T.);
#12960=ADVANCED_FACE('',(#1681),#1303,.T.);
#12961=ADVANCED_FACE('',(#1682,#1016,#1017,#1018,#1019,#1020,#1021,#1022,
#1023,#1024,#1025,#1026,#1027,#1028,#1029,#1030,#1031),#1304,.T.);
#13712=CLOSED_SHELL('',(#12912,#12913,#12914,#12915,#12916,#12917,#12918,
#12919,#12920,#12921,#12922,#12923,#12924,#12925,#12926,#12927,#12928,#12929,
#12930,#12931,#12932,#12933,#12934,#12935,#12936,#12937,#12938,#12939,#12940,
#12941,#12942,#12943,#12944,#12945,#12946,#12947,#12948,#12949,#12950,#12951,
#12952,#12953,#12954,#12955,#12956,#12957,#12958,#12959,#12960,#12961));
#14564=AXIS2_PLACEMENT_3D('',#20972,#16438,#16439);
#14565=AXIS2_PLACEMENT_3D('',#20973,#16440,#16441);
#14566=AXIS2_PLACEMENT_3D('',#20975,#16442,#16443);
#14567=AXIS2_PLACEMENT_3D('',#20978,#16445,#16446);
#14568=AXIS2_PLACEMENT_3D('',#20979,#16447,#16448);
#14569=AXIS2_PLACEMENT_3D('',#20980,#16449,#16450);
#14570=AXIS2_PLACEMENT_3D('',#20982,#16451,#16452);
#14571=AXIS2_PLACEMENT_3D('',#20985,#16454,#16455);
#14572=AXIS2_PLACEMENT_3D('',#20986,#16456,#16457);
#14573=AXIS2_PLACEMENT_3D('',#20987,#16458,#16459);
#14574=AXIS2_PLACEMENT_3D('',#20989,#16460,#16461);
#14575=AXIS2_PLACEMENT_3D('',#20992,#16463,#16464);
#14576=AXIS2_PLACEMENT_3D('',#20993,#16465,#16466);
#14577=AXIS2_PLACEMENT_3D('',#20994,#16467,#16468);
#14578=AXIS2_PLACEMENT_3D('',#20996,#16469,#16470);
#14579=AXIS2_PLACEMENT_3D('',#20999,#16472,#16473);
#14580=AXIS2_PLACEMENT_3D('',#21000,#16474,#16475);
#14581=AXIS2_PLACEMENT_3D('',#21001,#16476,#16477);
#14582=AXIS2_PLACEMENT_3D('',#21003,#16478,#16479);
#14583=AXIS2_PLACEMENT_3D('',#21006,#16481,#16482);
#14584=AXIS2_PLACEMENT_3D('',#21007,#16483,#16484);
#14585=AXIS2_PLACEMENT_3D('',#21008,#16485,#16486);
#14586=AXIS2_PLACEMENT_3D('',#21010,#16487,#16488);
#14587=AXIS2_PLACEMENT_3D('',#21013,#16490,#16491);
#14588=AXIS2_PLACEMENT_3D('',#21014,#16492,#16493);
#14589=AXIS2_PLACEMENT_3D('',#21015,#16494,#16495);
#14590=AXIS2_PLACEMENT_3D('',#21017,#16496,#16497);
#14591=AXIS2_PLACEMENT_3D('',#21020,#16499,#16500);
#14592=AXIS2_PLACEMENT_3D('',#21021,#16501,#16502);
#14593=AXIS2_PLACEMENT_3D('',#21022,#16503,#16504);
#14594=AXIS2_PLACEMENT_3D('',#21024,#16505,#16506);
#14595=AXIS2_PLACEMENT_3D('',#21027,#16508,#16509);
#14596=AXIS2_PLACEMENT_3D('',#21028,#16510,#16511);
#14597=AXIS2_PLACEMENT_3D('',#21029,#16512,#16513);
#14598=AXIS2_PLACEMENT_3D('',#21031,#16514,#16515);
#14599=AXIS2_PLACEMENT_3D('',#21034,#16517,#16518);
#14600=AXIS2_PLACEMENT_3D('',#21035,#16519,#16520);
#14601=AXIS2_PLACEMENT_3D('',#21036,#16521,#16522);
#14602=AXIS2_PLACEMENT_3D('',#21038,#16523,#16524);
#14603=AXIS2_PLACEMENT_3D('',#21041,#16526,#16527);
#14604=AXIS2_PLACEMENT_3D('',#21042,#16528,#16529);
#14605=AXIS2_PLACEMENT_3D('',#21043,#16530,#16531);
#14606=AXIS2_PLACEMENT_3D('',#21048,#16533,#16534);
#14607=AXIS2_PLACEMENT_3D('',#21051,#16536,#16537);
#14608=AXIS2_PLACEMENT_3D('',#21052,#16538,#16539);
#14609=AXIS2_PLACEMENT_3D('',#21057,#16541,#16542);
#14610=AXIS2_PLACEMENT_3D('',#21060,#16544,#16545);
#14611=AXIS2_PLACEMENT_3D('',#21061,#16546,#16547);
#14612=AXIS2_PLACEMENT_3D('',#21072,#16552,#16553);
#14613=AXIS2_PLACEMENT_3D('',#21076,#16555,#16556);
#14614=AXIS2_PLACEMENT_3D('',#21080,#16558,#16559);
#14615=AXIS2_PLACEMENT_3D('',#21084,#16561,#16562);
#14616=AXIS2_PLACEMENT_3D('',#21088,#16564,#16565);
#14617=AXIS2_PLACEMENT_3D('',#21092,#16567,#16568);
#14618=AXIS2_PLACEMENT_3D('',#21096,#16572,#16573);
#14619=AXIS2_PLACEMENT_3D('',#21098,#16575,#16576);
#14620=AXIS2_PLACEMENT_3D('',#21100,#16578,#16579);
#14621=AXIS2_PLACEMENT_3D('',#21105,#16582,#16583);
#14622=AXIS2_PLACEMENT_3D('',#21106,#16584,#16585);
#14623=AXIS2_PLACEMENT_3D('',#21110,#16587,#16588);
#14624=AXIS2_PLACEMENT_3D('',#21112,#16590,#16591);
#14625=AXIS2_PLACEMENT_3D('',#21114,#16593,#16594);
#14626=AXIS2_PLACEMENT_3D('',#21116,#16596,#16597);
#14627=AXIS2_PLACEMENT_3D('',#21121,#16599,#16600);
#14628=AXIS2_PLACEMENT_3D('',#21126,#16603,#16604);
#14629=AXIS2_PLACEMENT_3D('',#21129,#16606,#16607);
#14630=AXIS2_PLACEMENT_3D('',#21130,#16608,#16609);
#14631=AXIS2_PLACEMENT_3D('',#21134,#16611,#16612);
#14632=AXIS2_PLACEMENT_3D('',#21136,#16614,#16615);
#14633=AXIS2_PLACEMENT_3D('',#21138,#16617,#16618);
#14634=AXIS2_PLACEMENT_3D('',#21140,#16620,#16621);
#14635=AXIS2_PLACEMENT_3D('',#21145,#16623,#16624);
#14636=AXIS2_PLACEMENT_3D('',#21150,#16627,#16628);
#14637=AXIS2_PLACEMENT_3D('',#21153,#16630,#16631);
#14638=AXIS2_PLACEMENT_3D('',#21154,#16632,#16633);
#14639=AXIS2_PLACEMENT_3D('',#21158,#16635,#16636);
#14640=AXIS2_PLACEMENT_3D('',#21160,#16638,#16639);
#14641=AXIS2_PLACEMENT_3D('',#21162,#16641,#16642);
#14642=AXIS2_PLACEMENT_3D('',#21164,#16644,#16645);
#14643=AXIS2_PLACEMENT_3D('',#21165,#16646,#16647);
#14644=AXIS2_PLACEMENT_3D('',#21166,#16648,#16649);
#14645=AXIS2_PLACEMENT_3D('',#21167,#16650,#16651);
#14646=AXIS2_PLACEMENT_3D('',#21168,#16652,#16653);
#14647=AXIS2_PLACEMENT_3D('',#21170,#16654,#16655);
#14648=AXIS2_PLACEMENT_3D('',#21173,#16657,#16658);
#14649=AXIS2_PLACEMENT_3D('',#21174,#16659,#16660);
#14650=AXIS2_PLACEMENT_3D('',#21175,#16661,#16662);
#14651=AXIS2_PLACEMENT_3D('',#21177,#16663,#16664);
#14652=AXIS2_PLACEMENT_3D('',#21180,#16666,#16667);
#14653=AXIS2_PLACEMENT_3D('',#21181,#16668,#16669);
#14654=AXIS2_PLACEMENT_3D('',#21182,#16670,#16671);
#14655=AXIS2_PLACEMENT_3D('',#21183,#16672,#16673);
#14656=AXIS2_PLACEMENT_3D('',#21184,#16674,#16675);
#14657=AXIS2_PLACEMENT_3D('',#21185,#16676,#16677);
#14658=AXIS2_PLACEMENT_3D('',#21186,#16678,#16679);
#14659=AXIS2_PLACEMENT_3D('',#21192,#16683,#16684);
#14660=AXIS2_PLACEMENT_3D('',#21196,#16687,#16688);
#14661=AXIS2_PLACEMENT_3D('',#21200,#16691,#16692);
#14662=AXIS2_PLACEMENT_3D('',#21202,#16694,#16695);
#16438=DIRECTION('axis',(0.,0.,1.));
#16439=DIRECTION('refdir',(1.,0.,0.));
#16440=DIRECTION('center_axis',(0.,0.,1.));
#16441=DIRECTION('ref_axis',(1.,0.,0.));
#16442=DIRECTION('center_axis',(0.,0.,1.));
#16443=DIRECTION('ref_axis',(1.,0.,0.));
#16444=DIRECTION('',(0.,0.,1.));
#16445=DIRECTION('center_axis',(0.,0.,-1.));
#16446=DIRECTION('ref_axis',(1.,0.,0.));
#16447=DIRECTION('center_axis',(0.,0.,1.));
#16448=DIRECTION('ref_axis',(1.,0.,0.));
#16449=DIRECTION('center_axis',(0.,0.,1.));
#16450=DIRECTION('ref_axis',(1.,0.,0.));
#16451=DIRECTION('center_axis',(0.,0.,1.));
#16452=DIRECTION('ref_axis',(1.,0.,0.));
#16453=DIRECTION('',(0.,0.,1.));
#16454=DIRECTION('center_axis',(0.,0.,-1.));
#16455=DIRECTION('ref_axis',(1.,0.,0.));
#16456=DIRECTION('center_axis',(0.,0.,1.));
#16457=DIRECTION('ref_axis',(1.,0.,0.));
#16458=DIRECTION('center_axis',(0.,0.,1.));
#16459=DIRECTION('ref_axis',(1.,0.,0.));
#16460=DIRECTION('center_axis',(0.,0.,1.));
#16461=DIRECTION('ref_axis',(1.,0.,0.));
#16462=DIRECTION('',(0.,0.,1.));
#16463=DIRECTION('center_axis',(0.,0.,-1.));
#16464=DIRECTION('ref_axis',(1.,0.,0.));
#16465=DIRECTION('center_axis',(0.,0.,1.));
#16466=DIRECTION('ref_axis',(1.,0.,0.));
#16467=DIRECTION('center_axis',(0.,0.,1.));
#16468=DIRECTION('ref_axis',(1.,0.,0.));
#16469=DIRECTION('center_axis',(0.,0.,1.));
#16470=DIRECTION('ref_axis',(1.,0.,0.));
#16471=DIRECTION('',(0.,0.,1.));
#16472=DIRECTION('center_axis',(0.,0.,-1.));
#16473=DIRECTION('ref_axis',(1.,0.,0.));
#16474=DIRECTION('center_axis',(0.,0.,1.));
#16475=DIRECTION('ref_axis',(1.,0.,0.));
#16476=DIRECTION('center_axis',(0.,0.,1.));
#16477=DIRECTION('ref_axis',(1.,0.,0.));
#16478=DIRECTION('center_axis',(0.,0.,1.));
#16479=DIRECTION('ref_axis',(1.,0.,0.));
#16480=DIRECTION('',(0.,0.,1.));
#16481=DIRECTION('center_axis',(0.,0.,-1.));
#16482=DIRECTION('ref_axis',(1.,0.,0.));
#16483=DIRECTION('center_axis',(0.,0.,1.));
#16484=DIRECTION('ref_axis',(1.,0.,0.));
#16485=DIRECTION('center_axis',(0.,0.,1.));
#16486=DIRECTION('ref_axis',(1.,0.,0.));
#16487=DIRECTION('center_axis',(0.,0.,1.));
#16488=DIRECTION('ref_axis',(1.,0.,0.));
#16489=DIRECTION('',(0.,0.,1.));
#16490=DIRECTION('center_axis',(0.,0.,-1.));
#16491=DIRECTION('ref_axis',(1.,0.,0.));
#16492=DIRECTION('center_axis',(0.,0.,1.));
#16493=DIRECTION('ref_axis',(1.,0.,0.));
#16494=DIRECTION('center_axis',(0.,0.,1.));
#16495=DIRECTION('ref_axis',(1.,0.,0.));
#16496=DIRECTION('center_axis',(0.,0.,1.));
#16497=DIRECTION('ref_axis',(1.,0.,0.));
#16498=DIRECTION('',(0.,0.,1.));
#16499=DIRECTION('center_axis',(0.,0.,-1.));
#16500=DIRECTION('ref_axis',(1.,0.,0.));
#16501=DIRECTION('center_axis',(0.,0.,1.));
#16502=DIRECTION('ref_axis',(1.,0.,0.));
#16503=DIRECTION('center_axis',(0.,0.,1.));
#16504=DIRECTION('ref_axis',(1.,0.,0.));
#16505=DIRECTION('center_axis',(0.,0.,1.));
#16506=DIRECTION('ref_axis',(1.,0.,0.));
#16507=DIRECTION('',(0.,0.,1.));
#16508=DIRECTION('center_axis',(0.,0.,-1.));
#16509=DIRECTION('ref_axis',(1.,0.,0.));
#16510=DIRECTION('center_axis',(0.,0.,1.));
#16511=DIRECTION('ref_axis',(1.,0.,0.));
#16512=DIRECTION('center_axis',(0.,0.,1.));
#16513=DIRECTION('ref_axis',(1.,0.,0.));
#16514=DIRECTION('center_axis',(0.,0.,1.));
#16515=DIRECTION('ref_axis',(1.,0.,0.));
#16516=DIRECTION('',(0.,0.,1.));
#16517=DIRECTION('center_axis',(0.,0.,-1.));
#16518=DIRECTION('ref_axis',(1.,0.,0.));
#16519=DIRECTION('center_axis',(0.,0.,1.));
#16520=DIRECTION('ref_axis',(1.,0.,0.));
#16521=DIRECTION('center_axis',(0.,0.,1.));
#16522=DIRECTION('ref_axis',(1.,0.,0.));
#16523=DIRECTION('center_axis',(0.,0.,1.));
#16524=DIRECTION('ref_axis',(1.,0.,0.));
#16525=DIRECTION('',(0.,0.,1.));
#16526=DIRECTION('center_axis',(0.,0.,-1.));
#16527=DIRECTION('ref_axis',(1.,0.,0.));
#16528=DIRECTION('center_axis',(0.,0.,1.));
#16529=DIRECTION('ref_axis',(1.,0.,0.));
#16530=DIRECTION('center_axis',(0.,0.,1.));
#16531=DIRECTION('ref_axis',(-1.,-1.22464679914735E-16,0.));
#16532=DIRECTION('',(0.,0.,1.));
#16533=DIRECTION('center_axis',(0.,0.,1.));
#16534=DIRECTION('ref_axis',(1.,0.,0.));
#16535=DIRECTION('',(0.,0.,1.));
#16536=DIRECTION('center_axis',(0.,0.,-1.));
#16537=DIRECTION('ref_axis',(1.,0.,0.));
#16538=DIRECTION('center_axis',(0.,0.,1.));
#16539=DIRECTION('ref_axis',(1.,0.,0.));
#16540=DIRECTION('',(0.,0.,1.));
#16541=DIRECTION('center_axis',(0.,0.,-1.));
#16542=DIRECTION('ref_axis',(1.,0.,0.));
#16543=DIRECTION('',(0.,0.,1.));
#16544=DIRECTION('center_axis',(0.,0.,1.));
#16545=DIRECTION('ref_axis',(1.,0.,0.));
#16546=DIRECTION('center_axis',(0.,0.,1.));
#16547=DIRECTION('ref_axis',(1.,0.,0.));
#16548=DIRECTION('',(0.,-1.,0.));
#16549=DIRECTION('',(-1.,0.,0.));
#16550=DIRECTION('',(0.,1.,0.));
#16551=DIRECTION('',(1.,0.,0.));
#16552=DIRECTION('center_axis',(0.,0.,1.));
#16553=DIRECTION('ref_axis',(1.,0.,0.));
#16554=DIRECTION('',(1.,0.,0.));
#16555=DIRECTION('center_axis',(0.,0.,1.));
#16556=DIRECTION('ref_axis',(1.,0.,0.));
#16557=DIRECTION('',(-1.,0.,0.));
#16558=DIRECTION('center_axis',(0.,0.,1.));
#16559=DIRECTION('ref_axis',(1.,0.,0.));
#16560=DIRECTION('',(1.,0.,0.));
#16561=DIRECTION('center_axis',(0.,0.,1.));
#16562=DIRECTION('ref_axis',(1.,0.,0.));
#16563=DIRECTION('',(-1.,0.,0.));
#16564=DIRECTION('center_axis',(0.,0.,1.));
#16565=DIRECTION('ref_axis',(1.,0.,0.));
#16566=DIRECTION('',(1.,0.,0.));
#16567=DIRECTION('center_axis',(0.,0.,1.));
#16568=DIRECTION('ref_axis',(1.,0.,0.));
#16569=DIRECTION('',(-1.,0.,0.));
#16570=DIRECTION('',(1.,0.,0.));
#16571=DIRECTION('',(-1.,0.,0.));
#16572=DIRECTION('center_axis',(0.,1.,0.));
#16573=DIRECTION('ref_axis',(-1.,0.,0.));
#16574=DIRECTION('',(1.,0.,0.));
#16575=DIRECTION('center_axis',(0.,-1.,0.));
#16576=DIRECTION('ref_axis',(1.,0.,0.));
#16577=DIRECTION('',(-1.,0.,0.));
#16578=DIRECTION('center_axis',(0.,0.,1.));
#16579=DIRECTION('ref_axis',(-1.,-1.22464679914735E-16,0.));
#16580=DIRECTION('',(0.,0.,1.));
#16581=DIRECTION('',(0.,0.,1.));
#16582=DIRECTION('center_axis',(0.,0.,-1.));
#16583=DIRECTION('ref_axis',(1.,0.,0.));
#16584=DIRECTION('center_axis',(0.,0.,1.));
#16585=DIRECTION('ref_axis',(1.,0.,0.));
#16586=DIRECTION('',(0.,0.,1.));
#16587=DIRECTION('center_axis',(0.,0.,-1.));
#16588=DIRECTION('ref_axis',(1.,0.,0.));
#16589=DIRECTION('',(0.,0.,1.));
#16590=DIRECTION('center_axis',(0.,1.,0.));
#16591=DIRECTION('ref_axis',(-1.,0.,0.));
#16592=DIRECTION('',(1.,0.,0.));
#16593=DIRECTION('center_axis',(0.,-1.,0.));
#16594=DIRECTION('ref_axis',(1.,0.,0.));
#16595=DIRECTION('',(-1.,0.,0.));
#16596=DIRECTION('center_axis',(0.,0.,1.));
#16597=DIRECTION('ref_axis',(-1.,-1.22464679914735E-16,0.));
#16598=DIRECTION('',(0.,0.,-1.));
#16599=DIRECTION('center_axis',(0.,0.,-1.));
#16600=DIRECTION('ref_axis',(1.,0.,0.));
#16601=DIRECTION('',(0.,0.,1.));
#16602=DIRECTION('',(0.,0.,1.));
#16603=DIRECTION('center_axis',(0.,0.,-1.));
#16604=DIRECTION('ref_axis',(1.,0.,0.));
#16605=DIRECTION('',(0.,0.,1.));
#16606=DIRECTION('center_axis',(0.,0.,-1.));
#16607=DIRECTION('ref_axis',(1.,0.,0.));
#16608=DIRECTION('center_axis',(0.,0.,1.));
#16609=DIRECTION('ref_axis',(1.,0.,0.));
#16610=DIRECTION('',(0.,0.,1.));
#16611=DIRECTION('center_axis',(0.,0.,-1.));
#16612=DIRECTION('ref_axis',(1.,0.,0.));
#16613=DIRECTION('',(0.,0.,1.));
#16614=DIRECTION('center_axis',(0.,1.,0.));
#16615=DIRECTION('ref_axis',(-1.,0.,0.));
#16616=DIRECTION('',(1.,0.,0.));
#16617=DIRECTION('center_axis',(0.,-1.,0.));
#16618=DIRECTION('ref_axis',(1.,0.,0.));
#16619=DIRECTION('',(-1.,0.,0.));
#16620=DIRECTION('center_axis',(0.,0.,1.));
#16621=DIRECTION('ref_axis',(-1.,-1.22464679914735E-16,0.));
#16622=DIRECTION('',(0.,0.,-1.));
#16623=DIRECTION('center_axis',(0.,0.,-1.));
#16624=DIRECTION('ref_axis',(1.,0.,0.));
#16625=DIRECTION('',(0.,0.,1.));
#16626=DIRECTION('',(0.,0.,1.));
#16627=DIRECTION('center_axis',(0.,0.,-1.));
#16628=DIRECTION('ref_axis',(1.,0.,0.));
#16629=DIRECTION('',(0.,0.,1.));
#16630=DIRECTION('center_axis',(0.,0.,-1.));
#16631=DIRECTION('ref_axis',(1.,0.,0.));
#16632=DIRECTION('center_axis',(0.,0.,1.));
#16633=DIRECTION('ref_axis',(1.,0.,0.));
#16634=DIRECTION('',(0.,0.,1.));
#16635=DIRECTION('center_axis',(0.,0.,-1.));
#16636=DIRECTION('ref_axis',(1.,0.,0.));
#16637=DIRECTION('',(0.,0.,1.));
#16638=DIRECTION('center_axis',(0.,1.,0.));
#16639=DIRECTION('ref_axis',(-1.,0.,0.));
#16640=DIRECTION('',(1.,0.,0.));
#16641=DIRECTION('center_axis',(0.,-1.,0.));
#16642=DIRECTION('ref_axis',(1.,0.,0.));
#16643=DIRECTION('',(-1.,0.,0.));
#16644=DIRECTION('center_axis',(0.,0.,1.));
#16645=DIRECTION('ref_axis',(-1.,5.66553889764798E-16,0.));
#16646=DIRECTION('center_axis',(0.,0.,-1.));
#16647=DIRECTION('ref_axis',(1.,0.,0.));
#16648=DIRECTION('center_axis',(0.,0.,1.));
#16649=DIRECTION('ref_axis',(1.,0.,0.));
#16650=DIRECTION('center_axis',(0.,0.,1.));
#16651=DIRECTION('ref_axis',(1.,0.,0.));
#16652=DIRECTION('center_axis',(0.,0.,1.));
#16653=DIRECTION('ref_axis',(1.,0.,0.));
#16654=DIRECTION('center_axis',(0.,0.,1.));
#16655=DIRECTION('ref_axis',(1.,0.,0.));
#16656=DIRECTION('',(0.,0.,1.));
#16657=DIRECTION('center_axis',(0.,0.,-1.));
#16658=DIRECTION('ref_axis',(1.,0.,0.));
#16659=DIRECTION('center_axis',(0.,0.,1.));
#16660=DIRECTION('ref_axis',(1.,0.,0.));
#16661=DIRECTION('center_axis',(0.,0.,1.));
#16662=DIRECTION('ref_axis',(1.,0.,0.));
#16663=DIRECTION('center_axis',(0.,0.,1.));
#16664=DIRECTION('ref_axis',(1.,0.,0.));
#16665=DIRECTION('',(0.,0.,1.));
#16666=DIRECTION('center_axis',(0.,0.,-1.));
#16667=DIRECTION('ref_axis',(1.,0.,0.));
#16668=DIRECTION('center_axis',(0.,0.,1.));
#16669=DIRECTION('ref_axis',(1.,0.,0.));
#16670=DIRECTION('center_axis',(0.,0.,1.));
#16671=DIRECTION('ref_axis',(-1.,-3.21624529935327E-16,0.));
#16672=DIRECTION('center_axis',(0.,0.,-1.));
#16673=DIRECTION('ref_axis',(1.,0.,0.));
#16674=DIRECTION('center_axis',(0.,0.,1.));
#16675=DIRECTION('ref_axis',(1.,0.,0.));
#16676=DIRECTION('center_axis',(0.,0.,1.));
#16677=DIRECTION('ref_axis',(1.,0.,0.));
#16678=DIRECTION('center_axis',(0.,1.,0.));
#16679=DIRECTION('ref_axis',(-1.,0.,0.));
#16680=DIRECTION('',(0.,0.,1.));
#16681=DIRECTION('',(-1.,0.,0.));
#16682=DIRECTION('',(0.,0.,1.));
#16683=DIRECTION('center_axis',(1.,0.,0.));
#16684=DIRECTION('ref_axis',(0.,1.,0.));
#16685=DIRECTION('',(0.,1.,0.));
#16686=DIRECTION('',(0.,0.,1.));
#16687=DIRECTION('center_axis',(0.,-1.,0.));
#16688=DIRECTION('ref_axis',(1.,0.,0.));
#16689=DIRECTION('',(1.,0.,0.));
#16690=DIRECTION('',(0.,0.,1.));
#16691=DIRECTION('center_axis',(-1.,0.,0.));
#16692=DIRECTION('ref_axis',(0.,-1.,0.));
#16693=DIRECTION('',(0.,-1.,0.));
#16694=DIRECTION('center_axis',(0.,0.,1.));
#16695=DIRECTION('ref_axis',(1.,0.,0.));
#20972=CARTESIAN_POINT('',(0.,0.,0.));
#20973=CARTESIAN_POINT('Origin',(-1.5,8.5,-0.9));
#20974=CARTESIAN_POINT('',(-1.665,8.5,-0.9));
#20975=CARTESIAN_POINT('Origin',(-1.5,8.5,-0.9));
#20976=CARTESIAN_POINT('',(-1.665,8.5,0.));
#20977=CARTESIAN_POINT('',(-1.665,8.5,-0.9));
#20978=CARTESIAN_POINT('Origin',(-1.5,8.5,0.));
#20979=CARTESIAN_POINT('Origin',(-1.5,8.5,-0.9));
#20980=CARTESIAN_POINT('Origin',(-1.5,4.5,-0.9));
#20981=CARTESIAN_POINT('',(-1.665,4.5,-0.9));
#20982=CARTESIAN_POINT('Origin',(-1.5,4.5,-0.9));
#20983=CARTESIAN_POINT('',(-1.665,4.5,0.));
#20984=CARTESIAN_POINT('',(-1.665,4.5,-0.9));
#20985=CARTESIAN_POINT('Origin',(-1.5,4.5,0.));
#20986=CARTESIAN_POINT('Origin',(-1.5,4.5,-0.9));
#20987=CARTESIAN_POINT('Origin',(12.7709100301812,41.5,-1.1));
#20988=CARTESIAN_POINT('',(12.5609100301812,41.5,-1.1));
#20989=CARTESIAN_POINT('Origin',(12.7709100301812,41.5,-1.1));
#20990=CARTESIAN_POINT('',(12.5609100301812,41.5,0.));
#20991=CARTESIAN_POINT('',(12.5609100301812,41.5,-1.1));
#20992=CARTESIAN_POINT('Origin',(12.7709100301812,41.5,0.));
#20993=CARTESIAN_POINT('Origin',(12.7709100301812,41.5,-1.1));
#20994=CARTESIAN_POINT('Origin',(12.7709100301812,38.5,-1.1));
#20995=CARTESIAN_POINT('',(12.5609100301812,38.5,-1.1));
#20996=CARTESIAN_POINT('Origin',(12.7709100301812,38.5,-1.1));
#20997=CARTESIAN_POINT('',(12.5609100301812,38.5,0.));
#20998=CARTESIAN_POINT('',(12.5609100301812,38.5,-1.1));
#20999=CARTESIAN_POINT('Origin',(12.7709100301812,38.5,0.));
#21000=CARTESIAN_POINT('Origin',(12.7709100301812,38.5,-1.1));
#21001=CARTESIAN_POINT('Origin',(1.17091003018116,41.5,-1.1));
#21002=CARTESIAN_POINT('',(0.960910030181156,41.5,-1.1));
#21003=CARTESIAN_POINT('Origin',(1.17091003018116,41.5,-1.1));
#21004=CARTESIAN_POINT('',(0.960910030181156,41.5,0.));
#21005=CARTESIAN_POINT('',(0.960910030181156,41.5,-1.1));
#21006=CARTESIAN_POINT('Origin',(1.17091003018116,41.5,0.));
#21007=CARTESIAN_POINT('Origin',(1.17091003018116,41.5,-1.1));
#21008=CARTESIAN_POINT('Origin',(1.17091003018116,38.5,-1.1));
#21009=CARTESIAN_POINT('',(0.960910030181156,38.5,-1.1));
#21010=CARTESIAN_POINT('Origin',(1.17091003018116,38.5,-1.1));
#21011=CARTESIAN_POINT('',(0.960910030181156,38.5,0.));
#21012=CARTESIAN_POINT('',(0.960910030181156,38.5,-1.1));
#21013=CARTESIAN_POINT('Origin',(1.17091003018116,38.5,0.));
#21014=CARTESIAN_POINT('Origin',(1.17091003018116,38.5,-1.1));
#21015=CARTESIAN_POINT('Origin',(12.7709100301812,5.5,-1.1));
#21016=CARTESIAN_POINT('',(12.5609100301812,5.5,-1.1));
#21017=CARTESIAN_POINT('Origin',(12.7709100301812,5.5,-1.1));
#21018=CARTESIAN_POINT('',(12.5609100301812,5.5,0.));
#21019=CARTESIAN_POINT('',(12.5609100301812,5.5,-1.1));
#21020=CARTESIAN_POINT('Origin',(12.7709100301812,5.5,0.));
#21021=CARTESIAN_POINT('Origin',(12.7709100301812,5.5,-1.1));
#21022=CARTESIAN_POINT('Origin',(12.7709100301812,2.5,-1.1));
#21023=CARTESIAN_POINT('',(12.5609100301812,2.5,-1.1));
#21024=CARTESIAN_POINT('Origin',(12.7709100301812,2.5,-1.1));
#21025=CARTESIAN_POINT('',(12.5609100301812,2.5,0.));
#21026=CARTESIAN_POINT('',(12.5609100301812,2.5,-1.1));
#21027=CARTESIAN_POINT('Origin',(12.7709100301812,2.5,0.));
#21028=CARTESIAN_POINT('Origin',(12.7709100301812,2.5,-1.1));
#21029=CARTESIAN_POINT('Origin',(1.17091003018116,5.5,-1.1));
#21030=CARTESIAN_POINT('',(0.960910030181156,5.5,-1.1));
#21031=CARTESIAN_POINT('Origin',(1.17091003018116,5.5,-1.1));
#21032=CARTESIAN_POINT('',(0.960910030181156,5.5,0.));
#21033=CARTESIAN_POINT('',(0.960910030181156,5.5,-1.1));
#21034=CARTESIAN_POINT('Origin',(1.17091003018116,5.5,0.));
#21035=CARTESIAN_POINT('Origin',(1.17091003018116,5.5,-1.1));
#21036=CARTESIAN_POINT('Origin',(1.17091003018116,2.5,-1.1));
#21037=CARTESIAN_POINT('',(0.960910030181156,2.5,-1.1));
#21038=CARTESIAN_POINT('Origin',(1.17091003018116,2.5,-1.1));
#21039=CARTESIAN_POINT('',(0.960910030181156,2.5,0.));
#21040=CARTESIAN_POINT('',(0.960910030181156,2.5,-1.1));
#21041=CARTESIAN_POINT('Origin',(1.17091003018116,2.5,0.));
#21042=CARTESIAN_POINT('Origin',(1.17091003018116,2.5,-1.1));
#21043=CARTESIAN_POINT('Origin',(8.77091003018116,1.,-1.3));
#21044=CARTESIAN_POINT('',(8.77091003018116,0.775,-1.2));
#21045=CARTESIAN_POINT('',(8.77091003018116,0.775,0.));
#21046=CARTESIAN_POINT('',(8.77091003018116,0.775,-1.3));
#21047=CARTESIAN_POINT('',(8.77091003018116,1.225,-1.2));
#21048=CARTESIAN_POINT('Origin',(8.77091003018116,1.,-1.2));
#21049=CARTESIAN_POINT('',(8.77091003018116,1.225,0.));
#21050=CARTESIAN_POINT('',(8.77091003018116,1.225,-1.3));
#21051=CARTESIAN_POINT('Origin',(8.77091003018116,1.,0.));
#21052=CARTESIAN_POINT('Origin',(10.7709100301812,1.,-1.3));
#21053=CARTESIAN_POINT('',(10.7709100301812,0.775,-1.2));
#21054=CARTESIAN_POINT('',(10.7709100301812,0.775,0.));
#21055=CARTESIAN_POINT('',(10.7709100301812,0.775,-1.3));
#21056=CARTESIAN_POINT('',(10.7709100301812,1.225,0.));
#21057=CARTESIAN_POINT('Origin',(10.7709100301812,1.,0.));
#21058=CARTESIAN_POINT('',(10.7709100301812,1.225,-1.2));
#21059=CARTESIAN_POINT('',(10.7709100301812,1.225,-1.3));
#21060=CARTESIAN_POINT('Origin',(10.7709100301812,1.,-1.2));
#21061=CARTESIAN_POINT('Origin',(5.25,19.,-1.2));
#21062=CARTESIAN_POINT('',(-4.,44.5,-1.2));
#21063=CARTESIAN_POINT('',(-4.,-6.5,-1.2));
#21064=CARTESIAN_POINT('',(-4.,44.5,-1.2));
#21065=CARTESIAN_POINT('',(14.5,44.5,-1.2));
#21066=CARTESIAN_POINT('',(14.5,44.5,-1.2));
#21067=CARTESIAN_POINT('',(14.5,-6.5,-1.2));
#21068=CARTESIAN_POINT('',(14.5,-6.5,-1.2));
#21069=CARTESIAN_POINT('',(-4.,-6.5,-1.2));
#21070=CARTESIAN_POINT('',(8.77091003018116,-0.775,-1.2));
#21071=CARTESIAN_POINT('',(8.77091003018116,-1.225,-1.2));
#21072=CARTESIAN_POINT('Origin',(8.77091003018116,-1.,-1.2));
#21073=CARTESIAN_POINT('',(10.7709100301812,-1.225,-1.2));
#21074=CARTESIAN_POINT('',(7.01045501509058,-1.225,-1.2));
#21075=CARTESIAN_POINT('',(10.7709100301812,-0.775,-1.2));
#21076=CARTESIAN_POINT('Origin',(10.7709100301812,-1.,-1.2));
#21077=CARTESIAN_POINT('',(8.01045501509058,-0.774999999999999,-1.2));
#21078=CARTESIAN_POINT('',(3.17091003018116,-0.775,-1.2));
#21079=CARTESIAN_POINT('',(3.17091003018116,-1.225,-1.2));
#21080=CARTESIAN_POINT('Origin',(3.17091003018116,-1.,-1.2));
#21081=CARTESIAN_POINT('',(5.17091003018116,-1.225,-1.2));
#21082=CARTESIAN_POINT('',(4.21045501509058,-1.225,-1.2));
#21083=CARTESIAN_POINT('',(5.17091003018116,-0.775,-1.2));
#21084=CARTESIAN_POINT('Origin',(5.17091003018116,-1.,-1.2));
#21085=CARTESIAN_POINT('',(5.21045501509058,-0.774999999999999,-1.2));
#21086=CARTESIAN_POINT('',(3.17091003018116,1.225,-1.2));
#21087=CARTESIAN_POINT('',(3.17091003018116,0.775,-1.2));
#21088=CARTESIAN_POINT('Origin',(3.17091003018116,1.,-1.2));
#21089=CARTESIAN_POINT('',(5.17091003018116,0.775,-1.2));
#21090=CARTESIAN_POINT('',(4.21045501509058,0.774999999999999,-1.2));
#21091=CARTESIAN_POINT('',(5.17091003018116,1.225,-1.2));
#21092=CARTESIAN_POINT('Origin',(5.17091003018116,1.,-1.2));
#21093=CARTESIAN_POINT('',(5.21045501509058,1.225,-1.2));
#21094=CARTESIAN_POINT('',(7.01045501509058,0.774999999999999,-1.2));
#21095=CARTESIAN_POINT('',(8.01045501509058,1.225,-1.2));
#21096=CARTESIAN_POINT('Origin',(10.7709100301812,1.225,-1.3));
#21097=CARTESIAN_POINT('',(8.01045501509058,1.225,0.));
#21098=CARTESIAN_POINT('Origin',(8.77091003018116,0.775,-1.3));
#21099=CARTESIAN_POINT('',(7.01045501509058,0.774999999999999,0.));
#21100=CARTESIAN_POINT('Origin',(8.77091003018116,-1.,-1.3));
#21101=CARTESIAN_POINT('',(8.77091003018116,-1.225,0.));
#21102=CARTESIAN_POINT('',(8.77091003018116,-1.225,-1.3));
#21103=CARTESIAN_POINT('',(8.77091003018116,-0.775,0.));
#21104=CARTESIAN_POINT('',(8.77091003018116,-0.775,-1.3));
#21105=CARTESIAN_POINT('Origin',(8.77091003018116,-1.,0.));
#21106=CARTESIAN_POINT('Origin',(10.7709100301812,-1.,-1.3));
#21107=CARTESIAN_POINT('',(10.7709100301812,-1.225,0.));
#21108=CARTESIAN_POINT('',(10.7709100301812,-1.225,-1.3));
#21109=CARTESIAN_POINT('',(10.7709100301812,-0.775,0.));
#21110=CARTESIAN_POINT('Origin',(10.7709100301812,-1.,0.));
#21111=CARTESIAN_POINT('',(10.7709100301812,-0.775,-1.3));
#21112=CARTESIAN_POINT('Origin',(10.7709100301812,-0.775,-1.3));
#21113=CARTESIAN_POINT('',(8.01045501509058,-0.774999999999999,0.));
#21114=CARTESIAN_POINT('Origin',(8.77091003018116,-1.225,-1.3));
#21115=CARTESIAN_POINT('',(7.01045501509058,-1.225,0.));
#21116=CARTESIAN_POINT('Origin',(3.17091003018116,1.,-1.3));
#21117=CARTESIAN_POINT('',(2.9539109773241,0.940532268757414,0.));
#21118=CARTESIAN_POINT('',(2.9539109773241,0.940532268757414,-1.1));
#21119=CARTESIAN_POINT('',(2.9539109773241,0.940532268757414,-1.3));
#21120=CARTESIAN_POINT('',(3.17091003018116,0.775,0.));
#21121=CARTESIAN_POINT('Origin',(3.17091003018116,1.,0.));
#21122=CARTESIAN_POINT('',(3.17091003018116,0.775,-1.3));
#21123=CARTESIAN_POINT('',(3.17091003018116,1.225,0.));
#21124=CARTESIAN_POINT('',(3.17091003018116,1.225,-1.3));
#21125=CARTESIAN_POINT('',(2.9539109773241,1.05946773124259,0.));
#21126=CARTESIAN_POINT('Origin',(3.17091003018116,1.,0.));
#21127=CARTESIAN_POINT('',(2.9539109773241,1.05946773124259,-1.1));
#21128=CARTESIAN_POINT('',(2.9539109773241,1.05946773124259,-1.3));
#21129=CARTESIAN_POINT('Origin',(3.17091003018116,1.,-1.1));
#21130=CARTESIAN_POINT('Origin',(5.17091003018116,1.,-1.3));
#21131=CARTESIAN_POINT('',(5.17091003018116,0.775,0.));
#21132=CARTESIAN_POINT('',(5.17091003018116,0.775,-1.3));
#21133=CARTESIAN_POINT('',(5.17091003018116,1.225,0.));
#21134=CARTESIAN_POINT('Origin',(5.17091003018116,1.,0.));
#21135=CARTESIAN_POINT('',(5.17091003018116,1.225,-1.3));
#21136=CARTESIAN_POINT('Origin',(5.17091003018116,1.225,-1.3));
#21137=CARTESIAN_POINT('',(5.21045501509058,1.225,0.));
#21138=CARTESIAN_POINT('Origin',(3.17091003018116,0.775,-1.3));
#21139=CARTESIAN_POINT('',(4.21045501509058,0.774999999999999,0.));
#21140=CARTESIAN_POINT('Origin',(3.17091003018116,-1.,-1.3));
#21141=CARTESIAN_POINT('',(2.9539109773241,-1.05946773124259,0.));
#21142=CARTESIAN_POINT('',(2.9539109773241,-1.05946773124259,-1.1));
#21143=CARTESIAN_POINT('',(2.9539109773241,-1.05946773124259,-1.3));
#21144=CARTESIAN_POINT('',(3.17091003018116,-1.225,0.));
#21145=CARTESIAN_POINT('Origin',(3.17091003018116,-1.,0.));
#21146=CARTESIAN_POINT('',(3.17091003018116,-1.225,-1.3));
#21147=CARTESIAN_POINT('',(3.17091003018116,-0.775,0.));
#21148=CARTESIAN_POINT('',(3.17091003018116,-0.775,-1.3));
#21149=CARTESIAN_POINT('',(2.9539109773241,-0.940532268757414,0.));
#21150=CARTESIAN_POINT('Origin',(3.17091003018116,-1.,0.));
#21151=CARTESIAN_POINT('',(2.9539109773241,-0.940532268757414,-1.1));
#21152=CARTESIAN_POINT('',(2.9539109773241,-0.940532268757414,-1.3));
#21153=CARTESIAN_POINT('Origin',(3.17091003018116,-1.,-1.1));
#21154=CARTESIAN_POINT('Origin',(5.17091003018116,-1.,-1.3));
#21155=CARTESIAN_POINT('',(5.17091003018116,-1.225,0.));
#21156=CARTESIAN_POINT('',(5.17091003018116,-1.225,-1.3));
#21157=CARTESIAN_POINT('',(5.17091003018116,-0.775,0.));
#21158=CARTESIAN_POINT('Origin',(5.17091003018116,-1.,0.));
#21159=CARTESIAN_POINT('',(5.17091003018116,-0.775,-1.3));
#21160=CARTESIAN_POINT('Origin',(5.17091003018116,-0.775,-1.3));
#21161=CARTESIAN_POINT('',(5.21045501509058,-0.774999999999999,0.));
#21162=CARTESIAN_POINT('Origin',(3.17091003018116,-1.225,-1.3));
#21163=CARTESIAN_POINT('',(4.21045501509058,-1.225,0.));
#21164=CARTESIAN_POINT('Origin',(2.8,-1.,-1.1));
#21165=CARTESIAN_POINT('Origin',(2.8,-1.,0.));
#21166=CARTESIAN_POINT('Origin',(2.8,-1.,-1.1));
#21167=CARTESIAN_POINT('Origin',(2.8,-1.,-1.1));
#21168=CARTESIAN_POINT('Origin',(-2.8,1.,-1.1));
#21169=CARTESIAN_POINT('',(-2.965,1.,-1.1));
#21170=CARTESIAN_POINT('Origin',(-2.8,1.,-1.1));
#21171=CARTESIAN_POINT('',(-2.965,1.,0.));
#21172=CARTESIAN_POINT('',(-2.965,1.,-1.1));
#21173=CARTESIAN_POINT('Origin',(-2.8,1.,0.));
#21174=CARTESIAN_POINT('Origin',(-2.8,1.,-1.1));
#21175=CARTESIAN_POINT('Origin',(-2.8,-1.,-1.1));
#21176=CARTESIAN_POINT('',(-2.965,-1.,-1.1));
#21177=CARTESIAN_POINT('Origin',(-2.8,-1.,-1.1));
#21178=CARTESIAN_POINT('',(-2.965,-1.,0.));
#21179=CARTESIAN_POINT('',(-2.965,-1.,-1.1));
#21180=CARTESIAN_POINT('Origin',(-2.8,-1.,0.));
#21181=CARTESIAN_POINT('Origin',(-2.8,-1.,-1.1));
#21182=CARTESIAN_POINT('Origin',(2.8,1.,-1.1));
#21183=CARTESIAN_POINT('Origin',(2.8,1.,0.));
#21184=CARTESIAN_POINT('Origin',(2.8,1.,-1.1));
#21185=CARTESIAN_POINT('Origin',(2.8,1.,-1.1));
#21186=CARTESIAN_POINT('Origin',(14.5,44.5,-1.2));
#21187=CARTESIAN_POINT('',(-4.,44.5,0.));
#21188=CARTESIAN_POINT('',(-4.,44.5,-1.2));
#21189=CARTESIAN_POINT('',(14.5,44.5,0.));
#21190=CARTESIAN_POINT('',(14.5,44.5,0.));
#21191=CARTESIAN_POINT('',(14.5,44.5,-1.2));
#21192=CARTESIAN_POINT('Origin',(14.5,-6.5,-1.2));
#21193=CARTESIAN_POINT('',(14.5,-6.5,0.));
#21194=CARTESIAN_POINT('',(14.5,-6.5,0.));
#21195=CARTESIAN_POINT('',(14.5,-6.5,-1.2));
#21196=CARTESIAN_POINT('Origin',(-4.,-6.5,-1.2));
#21197=CARTESIAN_POINT('',(-4.,-6.5,0.));
#21198=CARTESIAN_POINT('',(-4.,-6.5,0.));
#21199=CARTESIAN_POINT('',(-4.,-6.5,-1.2));
#21200=CARTESIAN_POINT('Origin',(-4.,44.5,-1.2));
#21201=CARTESIAN_POINT('',(-4.,44.5,0.));
#21202=CARTESIAN_POINT('Origin',(5.25,19.,0.));
#26918=UNCERTAINTY_MEASURE_WITH_UNIT(LENGTH_MEASURE(0.001),#27070,
'DISTANCE_ACCURACY_VALUE',
'Maximum model space distance between geometric entities at asserted c
onnectivities');
#26992=UNCERTAINTY_MEASURE_WITH_UNIT(LENGTH_MEASURE(0.001),#27070,
'DISTANCE_ACCURACY_VALUE',
'Maximum model space distance between geometric entities at asserted c
onnectivities');
#26995=(
GEOMETRIC_REPRESENTATION_CONTEXT(3)
GLOBAL_UNCERTAINTY_ASSIGNED_CONTEXT((#26918))
GLOBAL_UNIT_ASSIGNED_CONTEXT((#27070,#27072,#27073))
REPRESENTATION_CONTEXT('','3D')
);
#27069=(
GEOMETRIC_REPRESENTATION_CONTEXT(3)
GLOBAL_UNCERTAINTY_ASSIGNED_CONTEXT((#26992))
GLOBAL_UNIT_ASSIGNED_CONTEXT((#27070,#27072,#27073))
REPRESENTATION_CONTEXT('','3D')
);
#27070=(
LENGTH_UNIT()
NAMED_UNIT(*)
SI_UNIT(.CENTI.,.METRE.)
);
#27072=(
NAMED_UNIT(*)
PLANE_ANGLE_UNIT()
SI_UNIT($,.RADIAN.)
);
#27073=(
NAMED_UNIT(*)
SI_UNIT($,.STERADIAN.)
SOLID_ANGLE_UNIT()
);
#27076=SHAPE_DEFINITION_REPRESENTATION(#27152,#27353);
#27152=PRODUCT_DEFINITION_SHAPE('',$,#27430);
#27353=SHAPE_REPRESENTATION('',(#14564),#26995);
#27427=PRODUCT_DEFINITION_CONTEXT('part definition',#27657,'design');
#27430=PRODUCT_DEFINITION('Base','Base',#27506,#27427);
#27506=PRODUCT_DEFINITION_FORMATION('',$,#27661);
#27657=APPLICATION_CONTEXT(
'Core Data for Automotive Mechanical Design Process');
#27658=PRODUCT_CONTEXT('part definition',#27657,'mechanical');
#27661=PRODUCT('Base','Base','Base',(#27658));
#27770=COLOUR_RGB('Dark Blue',0.08,0.2,0.34);
#27771=FILL_AREA_STYLE_COLOUR('',#27770);
#27772=FILL_AREA_STYLE('',(#27771));
#27773=SURFACE_STYLE_FILL_AREA(#27772);
#27774=SURFACE_SIDE_STYLE('',(#27773));
#27775=SURFACE_STYLE_USAGE(.BOTH.,#27774);
#27776=PRESENTATION_STYLE_ASSIGNMENT((#27775));
ENDSEC;
END-ISO-10303-21;
